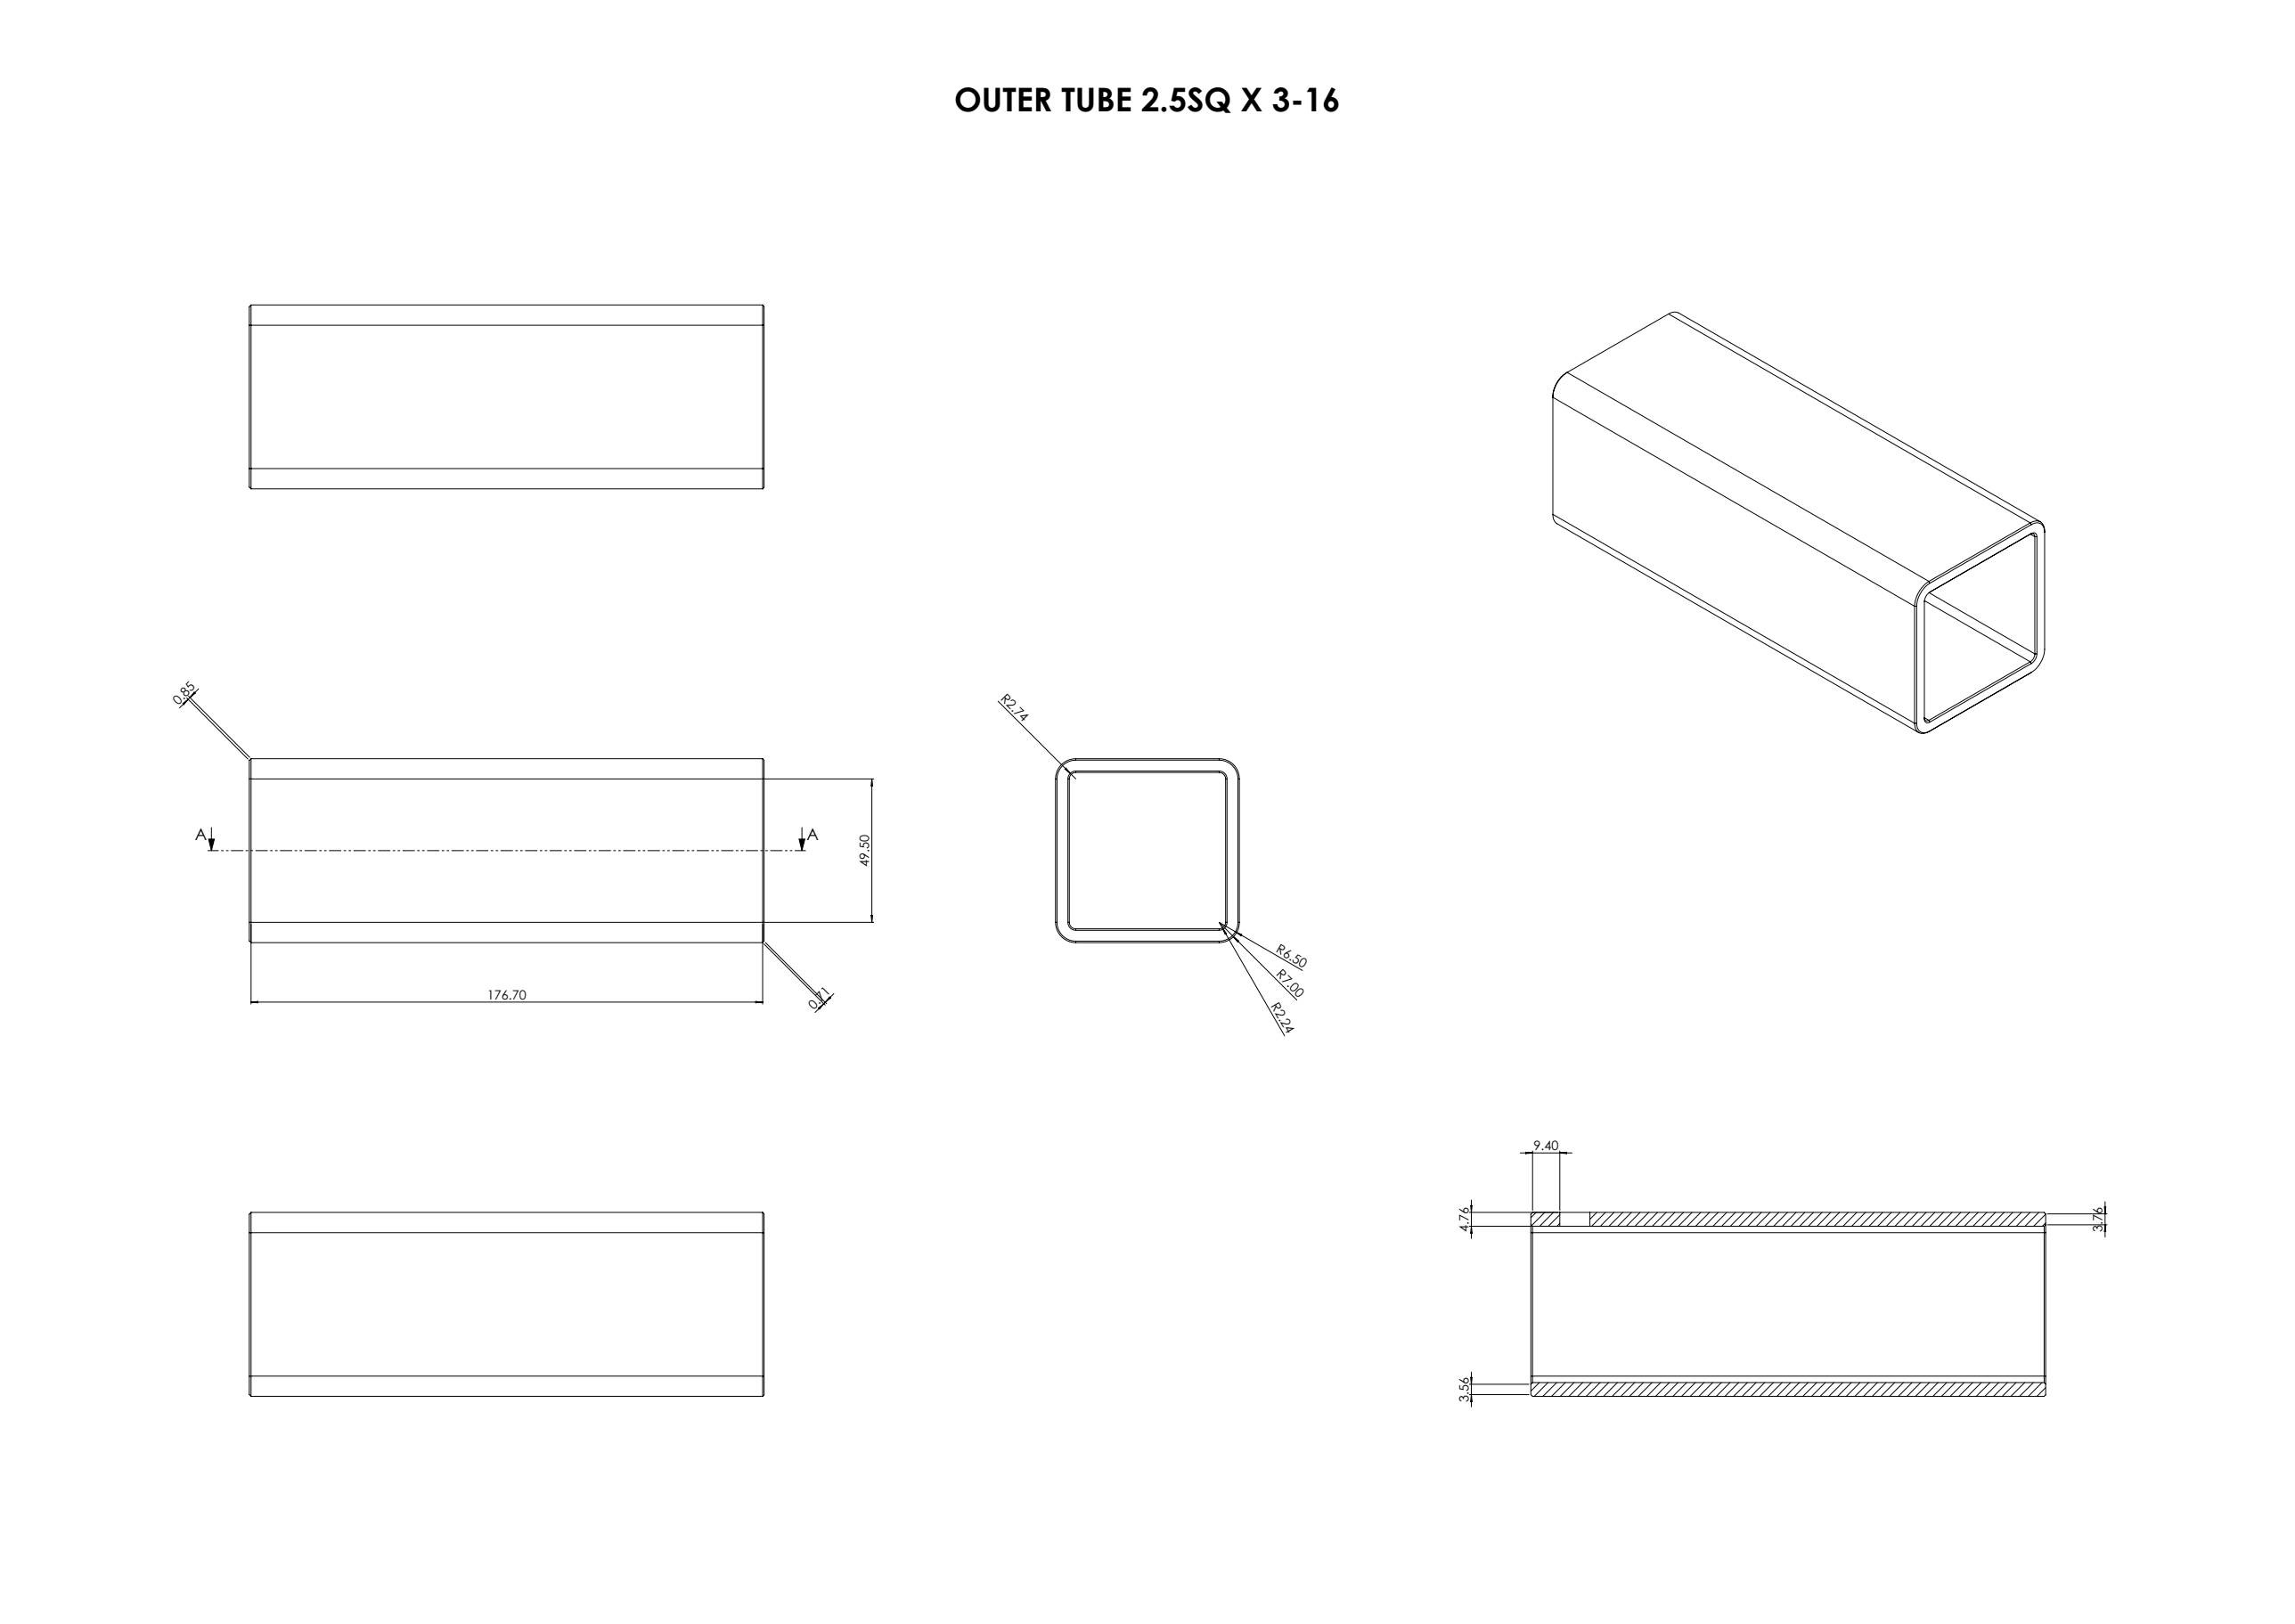
ISO-10303-21;
HEADER;
/* Generated by software containing ST-Developer
 * from STEP Tools, Inc. (www.steptools.com) 
 */

FILE_DESCRIPTION(
/* description */ (''),
/* implementation_level */ '2;1');

FILE_NAME(
/* name */ '01_Outer_Tube_2.5sq_x_3-16.step',
/* time_stamp */ '2026-10-25T01:30:15-07:00',
/* author */ (''),
/* organization */ (''),
/* preprocessor_version */ 'ST-DEVELOPER v20.2',
/* originating_system */ 'Autodesk Translation Framework v15.15.0.0',
/* authorisation */ '');

FILE_SCHEMA (('AUTOMOTIVE_DESIGN { 1 0 10303 214 3 1 1 }'));
ENDSEC;

DATA;
#10=MECHANICAL_DESIGN_GEOMETRIC_PRESENTATION_REPRESENTATION('',(#563),#32309);
#535=SHAPE_REPRESENTATION_RELATIONSHIP('SRR','None',#32362,#549);
#549=ADVANCED_BREP_SHAPE_REPRESENTATION('',(#577),#32295);
#563=STYLED_ITEM('',(#32488),#577);
#577=MANIFOLD_SOLID_BREP('Body1',#13804);
#591=FACE_BOUND('',#2051,.T.);
#592=FACE_BOUND('',#2055,.T.);
#593=FACE_BOUND('',#2078,.T.);
#594=FACE_BOUND('',#2095,.T.);
#647=CYLINDRICAL_SURFACE('',#13991,2.2375);
#648=CYLINDRICAL_SURFACE('',#13995,2.23749999999999);
#649=CYLINDRICAL_SURFACE('',#14015,7.);
#650=CYLINDRICAL_SURFACE('',#14018,7.);
#651=CYLINDRICAL_SURFACE('',#14035,7.);
#652=CYLINDRICAL_SURFACE('',#14051,2.23749999999998);
#653=CYLINDRICAL_SURFACE('',#14052,5.2);
#654=CYLINDRICAL_SURFACE('',#14055,2.2375);
#655=CYLINDRICAL_SURFACE('',#14058,7.);
#773=CIRCLE('',#13977,2.73749999999998);
#774=CIRCLE('',#13978,2.23749999999999);
#775=CIRCLE('',#13981,2.7375);
#776=CIRCLE('',#13982,2.2375);
#777=CIRCLE('',#13985,2.7375);
#778=CIRCLE('',#13986,2.2375);
#779=CIRCLE('',#13989,2.73749999999998);
#780=CIRCLE('',#13990,2.23749999999998);
#781=CIRCLE('',#13992,2.2375);
#782=CIRCLE('',#13994,5.2);
#783=CIRCLE('',#13996,2.23749999999999);
#784=CIRCLE('',#13999,6.5);
#785=CIRCLE('',#14000,6.5);
#786=CIRCLE('',#14001,6.50000000000001);
#787=CIRCLE('',#14002,6.5);
#788=CIRCLE('',#14005,7.);
#789=CIRCLE('',#14008,7.);
#790=CIRCLE('',#14011,7.);
#791=CIRCLE('',#14014,7.);
#792=CIRCLE('',#14016,7.);
#793=CIRCLE('',#14019,7.);
#794=CIRCLE('',#14023,6.4);
#795=CIRCLE('',#14026,7.);
#796=CIRCLE('',#14027,6.40000000000001);
#797=CIRCLE('',#14030,7.);
#798=CIRCLE('',#14031,6.40000000000001);
#799=CIRCLE('',#14034,6.4);
#800=CIRCLE('',#14037,2.83749999999998);
#801=CIRCLE('',#14038,2.83749999999998);
#802=CIRCLE('',#14039,2.83750000000001);
#803=CIRCLE('',#14040,2.8375);
#804=CIRCLE('',#14045,2.2375);
#805=CIRCLE('',#14048,2.23749999999998);
#806=CIRCLE('',#14053,5.2);
#1097=CONICAL_SURFACE('',#13976,2.48749999999999,0.785398163397441);
#1098=CONICAL_SURFACE('',#13980,2.4875,0.785398163397441);
#1099=CONICAL_SURFACE('',#13984,2.4875,0.785398163397441);
#1100=CONICAL_SURFACE('',#13988,2.48749999999998,0.785398163397441);
#1101=CONICAL_SURFACE('',#14004,6.75,0.785398163397441);
#1102=CONICAL_SURFACE('',#14007,6.75,0.785398163397441);
#1103=CONICAL_SURFACE('',#14010,6.75000000000001,0.785398163397431);
#1104=CONICAL_SURFACE('',#14013,6.75,0.785398163397441);
#1105=CONICAL_SURFACE('',#14022,6.7,0.78539816339745);
#1106=CONICAL_SURFACE('',#14025,6.70000000000001,0.785398163397438);
#1107=CONICAL_SURFACE('',#14029,6.7,0.785398163397445);
#1108=CONICAL_SURFACE('',#14033,6.7,0.78539816339745);
#1109=CONICAL_SURFACE('',#14042,2.5375,0.78539816339745);
#1110=CONICAL_SURFACE('',#14044,2.5375,0.78539816339745);
#1111=CONICAL_SURFACE('',#14047,2.53749999999998,0.785398163397445);
#1112=CONICAL_SURFACE('',#14050,2.53749999999998,0.785398163397445);
#1242=FACE_OUTER_BOUND('',#2041,.T.);
#1243=FACE_OUTER_BOUND('',#2042,.T.);
#1244=FACE_OUTER_BOUND('',#2043,.T.);
#1245=FACE_OUTER_BOUND('',#2044,.T.);
#1246=FACE_OUTER_BOUND('',#2045,.T.);
#1247=FACE_OUTER_BOUND('',#2046,.T.);
#1248=FACE_OUTER_BOUND('',#2047,.T.);
#1249=FACE_OUTER_BOUND('',#2048,.T.);
#1250=FACE_OUTER_BOUND('',#2049,.T.);
#1251=FACE_OUTER_BOUND('',#2050,.T.);
#1252=FACE_OUTER_BOUND('',#2052,.T.);
#1253=FACE_OUTER_BOUND('',#2053,.T.);
#1254=FACE_OUTER_BOUND('',#2054,.T.);
#1255=FACE_OUTER_BOUND('',#2056,.T.);
#1256=FACE_OUTER_BOUND('',#2057,.T.);
#1257=FACE_OUTER_BOUND('',#2058,.T.);
#1258=FACE_OUTER_BOUND('',#2059,.T.);
#1259=FACE_OUTER_BOUND('',#2060,.T.);
#1260=FACE_OUTER_BOUND('',#2061,.T.);
#1261=FACE_OUTER_BOUND('',#2062,.T.);
#1262=FACE_OUTER_BOUND('',#2063,.T.);
#1263=FACE_OUTER_BOUND('',#2064,.T.);
#1264=FACE_OUTER_BOUND('',#2065,.T.);
#1265=FACE_OUTER_BOUND('',#2066,.T.);
#1266=FACE_OUTER_BOUND('',#2067,.T.);
#1267=FACE_OUTER_BOUND('',#2068,.T.);
#1268=FACE_OUTER_BOUND('',#2069,.T.);
#1269=FACE_OUTER_BOUND('',#2070,.T.);
#1270=FACE_OUTER_BOUND('',#2071,.T.);
#1271=FACE_OUTER_BOUND('',#2072,.T.);
#1272=FACE_OUTER_BOUND('',#2073,.T.);
#1273=FACE_OUTER_BOUND('',#2074,.T.);
#1274=FACE_OUTER_BOUND('',#2075,.T.);
#1275=FACE_OUTER_BOUND('',#2076,.T.);
#1276=FACE_OUTER_BOUND('',#2077,.T.);
#1277=FACE_OUTER_BOUND('',#2079,.T.);
#1278=FACE_OUTER_BOUND('',#2080,.T.);
#1279=FACE_OUTER_BOUND('',#2081,.T.);
#1280=FACE_OUTER_BOUND('',#2082,.T.);
#1281=FACE_OUTER_BOUND('',#2083,.T.);
#1282=FACE_OUTER_BOUND('',#2084,.T.);
#1283=FACE_OUTER_BOUND('',#2085,.T.);
#1284=FACE_OUTER_BOUND('',#2086,.T.);
#1285=FACE_OUTER_BOUND('',#2087,.T.);
#1286=FACE_OUTER_BOUND('',#2088,.T.);
#1287=FACE_OUTER_BOUND('',#2089,.T.);
#1288=FACE_OUTER_BOUND('',#2090,.T.);
#1289=FACE_OUTER_BOUND('',#2091,.T.);
#1290=FACE_OUTER_BOUND('',#2092,.T.);
#1291=FACE_OUTER_BOUND('',#2093,.T.);
#1292=FACE_OUTER_BOUND('',#2094,.T.);
#2041=EDGE_LOOP('',(#8679,#8680,#8681,#8682));
#2042=EDGE_LOOP('',(#8683,#8684,#8685,#8686));
#2043=EDGE_LOOP('',(#8687,#8688,#8689,#8690));
#2044=EDGE_LOOP('',(#8691,#8692,#8693,#8694));
#2045=EDGE_LOOP('',(#8695,#8696,#8697,#8698));
#2046=EDGE_LOOP('',(#8699,#8700,#8701,#8702));
#2047=EDGE_LOOP('',(#8703,#8704,#8705,#8706));
#2048=EDGE_LOOP('',(#8707,#8708,#8709,#8710));
#2049=EDGE_LOOP('',(#8711,#8712,#8713,#8714));
#2050=EDGE_LOOP('',(#8715,#8716,#8717,#8718));
#2051=EDGE_LOOP('',(#8719));
#2052=EDGE_LOOP('',(#8720,#8721,#8722,#8723));
#2053=EDGE_LOOP('',(#8724,#8725,#8726,#8727));
#2054=EDGE_LOOP('',(#8728,#8729,#8730,#8731,#8732,#8733,#8734,#8735));
#2055=EDGE_LOOP('',(#8736,#8737,#8738,#8739,#8740,#8741,#8742,#8743));
#2056=EDGE_LOOP('',(#8744,#8745,#8746,#8747));
#2057=EDGE_LOOP('',(#8748,#8749,#8750,#8751));
#2058=EDGE_LOOP('',(#8752,#8753,#8754,#8755));
#2059=EDGE_LOOP('',(#8756,#8757,#8758,#8759));
#2060=EDGE_LOOP('',(#8760,#8761,#8762,#8763));
#2061=EDGE_LOOP('',(#8764,#8765,#8766,#8767));
#2062=EDGE_LOOP('',(#8768,#8769,#8770,#8771));
#2063=EDGE_LOOP('',(#8772,#8773,#8774,#8775));
#2064=EDGE_LOOP('',(#8776,#8777,#8778,#8779));
#2065=EDGE_LOOP('',(#8780,#8781,#8782,#8783));
#2066=EDGE_LOOP('',(#8784,#8785,#8786,#8787));
#2067=EDGE_LOOP('',(#8788,#8789,#8790,#8791));
#2068=EDGE_LOOP('',(#8792,#8793,#8794,#8795));
#2069=EDGE_LOOP('',(#8796,#8797,#8798,#8799));
#2070=EDGE_LOOP('',(#8800,#8801,#8802,#8803));
#2071=EDGE_LOOP('',(#8804,#8805,#8806,#8807));
#2072=EDGE_LOOP('',(#8808,#8809,#8810,#8811));
#2073=EDGE_LOOP('',(#8812,#8813,#8814,#8815));
#2074=EDGE_LOOP('',(#8816,#8817,#8818,#8819));
#2075=EDGE_LOOP('',(#8820,#8821,#8822,#8823));
#2076=EDGE_LOOP('',(#8824,#8825,#8826,#8827));
#2077=EDGE_LOOP('',(#8828,#8829,#8830,#8831,#8832,#8833,#8834,#8835));
#2078=EDGE_LOOP('',(#8836,#8837,#8838,#8839,#8840,#8841,#8842,#8843));
#2079=EDGE_LOOP('',(#8844,#8845,#8846,#8847));
#2080=EDGE_LOOP('',(#8848,#8849,#8850,#8851));
#2081=EDGE_LOOP('',(#8852,#8853,#8854,#8855));
#2082=EDGE_LOOP('',(#8856,#8857,#8858,#8859));
#2083=EDGE_LOOP('',(#8860,#8861,#8862,#8863));
#2084=EDGE_LOOP('',(#8864,#8865,#8866,#8867));
#2085=EDGE_LOOP('',(#8868,#8869,#8870,#8871));
#2086=EDGE_LOOP('',(#8872,#8873,#8874,#8875));
#2087=EDGE_LOOP('',(#8876,#8877,#8878,#8879));
#2088=EDGE_LOOP('',(#8880,#8881,#8882,#8883));
#2089=EDGE_LOOP('',(#8884,#8885,#8886,#8887));
#2090=EDGE_LOOP('',(#8888,#8889,#8890,#8891));
#2091=EDGE_LOOP('',(#8892,#8893,#8894,#8895));
#2092=EDGE_LOOP('',(#8896,#8897,#8898,#8899));
#2093=EDGE_LOOP('',(#8900,#8901,#8902,#8903));
#2094=EDGE_LOOP('',(#8904,#8905,#8906,#8907));
#2095=EDGE_LOOP('',(#8908));
#2896=LINE('',#18382,#4207);
#2897=LINE('',#18384,#4208);
#2898=LINE('',#18386,#4209);
#2899=LINE('',#18387,#4210);
#2900=LINE('',#18391,#4211);
#2901=LINE('',#18397,#4212);
#2902=LINE('',#18398,#4213);
#2903=LINE('',#18399,#4214);
#2904=LINE('',#18403,#4215);
#2905=LINE('',#18409,#4216);
#2906=LINE('',#18410,#4217);
#2907=LINE('',#18411,#4218);
#2908=LINE('',#18415,#4219);
#2909=LINE('',#18421,#4220);
#2910=LINE('',#18422,#4221);
#2911=LINE('',#18423,#4222);
#2912=LINE('',#18429,#4223);
#2913=LINE('',#18432,#4224);
#2914=LINE('',#18435,#4225);
#2915=LINE('',#18436,#4226);
#2916=LINE('',#18441,#4227);
#2917=LINE('',#18445,#4228);
#2918=LINE('',#18446,#4229);
#2919=LINE('',#18450,#4230);
#2920=LINE('',#18454,#4231);
#2921=LINE('',#18458,#4232);
#2922=LINE('',#18462,#4233);
#2923=LINE('',#18466,#4234);
#2924=LINE('',#18468,#4235);
#2925=LINE('',#18469,#4236);
#2926=LINE('',#18472,#4237);
#2927=LINE('',#18476,#4238);
#2928=LINE('',#18477,#4239);
#2929=LINE('',#18480,#4240);
#2930=LINE('',#18484,#4241);
#2931=LINE('',#18485,#4242);
#2932=LINE('',#18488,#4243);
#2933=LINE('',#18492,#4244);
#2934=LINE('',#18493,#4245);
#2935=LINE('',#18498,#4246);
#2936=LINE('',#18501,#4247);
#2937=LINE('',#18504,#4248);
#2938=LINE('',#18505,#4249);
#2939=LINE('',#18508,#4250);
#2940=LINE('',#18512,#4251);
#2941=LINE('',#18513,#4252);
#2942=LINE('',#18516,#4253);
#2943=LINE('',#18518,#4254);
#2944=LINE('',#18519,#4255);
#2945=LINE('',#18522,#4256);
#2946=LINE('',#18527,#4257);
#2947=LINE('',#18528,#4258);
#2948=LINE('',#18529,#4259);
#2949=LINE('',#18533,#4260);
#2950=LINE('',#18539,#4261);
#2951=LINE('',#18540,#4262);
#2952=LINE('',#18541,#4263);
#2953=LINE('',#18544,#4264);
#2954=LINE('',#18549,#4265);
#2955=LINE('',#18550,#4266);
#2956=LINE('',#18554,#4267);
#2957=LINE('',#18558,#4268);
#2958=LINE('',#18562,#4269);
#2959=LINE('',#18566,#4270);
#2960=LINE('',#18570,#4271);
#2961=LINE('',#18573,#4272);
#2962=LINE('',#18574,#4273);
#2963=LINE('',#18576,#4274);
#2964=LINE('',#18579,#4275);
#2965=LINE('',#18580,#4276);
#2966=LINE('',#18583,#4277);
#2967=LINE('',#18587,#4278);
#2968=LINE('',#18588,#4279);
#2969=LINE('',#18590,#4280);
#2970=LINE('',#18593,#4281);
#2971=LINE('',#18596,#4282);
#2972=LINE('',#18600,#4283);
#2973=LINE('',#18602,#4284);
#2974=LINE('',#18604,#4285);
#2975=LINE('',#18607,#4286);
#2976=LINE('',#18609,#4287);
#4207=VECTOR('',#15010,10.);
#4208=VECTOR('',#15011,10.);
#4209=VECTOR('',#15012,10.);
#4210=VECTOR('',#15013,10.);
#4211=VECTOR('',#15016,10.);
#4212=VECTOR('',#15023,10.);
#4213=VECTOR('',#15024,10.);
#4214=VECTOR('',#15025,10.);
#4215=VECTOR('',#15028,10.);
#4216=VECTOR('',#15035,10.);
#4217=VECTOR('',#15036,10.);
#4218=VECTOR('',#15037,10.);
#4219=VECTOR('',#15040,10.);
#4220=VECTOR('',#15047,10.);
#4221=VECTOR('',#15048,10.);
#4222=VECTOR('',#15049,10.);
#4223=VECTOR('',#15058,10.);
#4224=VECTOR('',#15061,10.);
#4225=VECTOR('',#15064,10.);
#4226=VECTOR('',#15065,10.);
#4227=VECTOR('',#15070,10.);
#4228=VECTOR('',#15075,10.);
#4229=VECTOR('',#15076,10.);
#4230=VECTOR('',#15079,10.);
#4231=VECTOR('',#15082,10.);
#4232=VECTOR('',#15085,10.);
#4233=VECTOR('',#15088,10.);
#4234=VECTOR('',#15093,10.);
#4235=VECTOR('',#15094,10.);
#4236=VECTOR('',#15095,10.);
#4237=VECTOR('',#15098,10.);
#4238=VECTOR('',#15103,10.);
#4239=VECTOR('',#15104,10.);
#4240=VECTOR('',#15107,10.);
#4241=VECTOR('',#15112,10.);
#4242=VECTOR('',#15113,10.);
#4243=VECTOR('',#15116,10.);
#4244=VECTOR('',#15121,10.);
#4245=VECTOR('',#15122,10.);
#4246=VECTOR('',#15129,10.);
#4247=VECTOR('',#15132,10.);
#4248=VECTOR('',#15135,10.);
#4249=VECTOR('',#15136,10.);
#4250=VECTOR('',#15139,10.);
#4251=VECTOR('',#15144,10.);
#4252=VECTOR('',#15145,10.);
#4253=VECTOR('',#15148,10.);
#4254=VECTOR('',#15149,10.);
#4255=VECTOR('',#15150,10.);
#4256=VECTOR('',#15153,10.);
#4257=VECTOR('',#15158,10.);
#4258=VECTOR('',#15159,10.);
#4259=VECTOR('',#15160,10.);
#4260=VECTOR('',#15163,10.);
#4261=VECTOR('',#15170,10.);
#4262=VECTOR('',#15171,10.);
#4263=VECTOR('',#15172,10.);
#4264=VECTOR('',#15175,10.);
#4265=VECTOR('',#15182,10.);
#4266=VECTOR('',#15183,10.);
#4267=VECTOR('',#15190,10.);
#4268=VECTOR('',#15193,10.);
#4269=VECTOR('',#15196,10.);
#4270=VECTOR('',#15199,10.);
#4271=VECTOR('',#15202,10.);
#4272=VECTOR('',#15207,10.);
#4273=VECTOR('',#15208,10.);
#4274=VECTOR('',#15211,10.);
#4275=VECTOR('',#15214,10.);
#4276=VECTOR('',#15215,10.);
#4277=VECTOR('',#15218,10.);
#4278=VECTOR('',#15223,10.);
#4279=VECTOR('',#15224,10.);
#4280=VECTOR('',#15227,10.);
#4281=VECTOR('',#15232,10.);
#4282=VECTOR('',#15237,10.);
#4283=VECTOR('',#15242,5.2);
#4284=VECTOR('',#15245,10.);
#4285=VECTOR('',#15248,10.);
#4286=VECTOR('',#15253,10.);
#4287=VECTOR('',#15256,10.);
#5518=VERTEX_POINT('',#18380);
#5519=VERTEX_POINT('',#18381);
#5520=VERTEX_POINT('',#18383);
#5521=VERTEX_POINT('',#18385);
#5522=VERTEX_POINT('',#18389);
#5523=VERTEX_POINT('',#18390);
#5524=VERTEX_POINT('',#18395);
#5525=VERTEX_POINT('',#18396);
#5526=VERTEX_POINT('',#18401);
#5527=VERTEX_POINT('',#18402);
#5528=VERTEX_POINT('',#18407);
#5529=VERTEX_POINT('',#18408);
#5530=VERTEX_POINT('',#18413);
#5531=VERTEX_POINT('',#18414);
#5532=VERTEX_POINT('',#18419);
#5533=VERTEX_POINT('',#18420);
#5534=VERTEX_POINT('',#18428);
#5535=VERTEX_POINT('',#18430);
#5536=VERTEX_POINT('',#18434);
#5537=VERTEX_POINT('',#18437);
#5538=VERTEX_POINT('',#18440);
#5539=VERTEX_POINT('',#18444);
#5540=VERTEX_POINT('',#18448);
#5541=VERTEX_POINT('',#18449);
#5542=VERTEX_POINT('',#18451);
#5543=VERTEX_POINT('',#18453);
#5544=VERTEX_POINT('',#18455);
#5545=VERTEX_POINT('',#18457);
#5546=VERTEX_POINT('',#18459);
#5547=VERTEX_POINT('',#18461);
#5548=VERTEX_POINT('',#18465);
#5549=VERTEX_POINT('',#18467);
#5550=VERTEX_POINT('',#18471);
#5551=VERTEX_POINT('',#18475);
#5552=VERTEX_POINT('',#18479);
#5553=VERTEX_POINT('',#18483);
#5554=VERTEX_POINT('',#18487);
#5555=VERTEX_POINT('',#18491);
#5556=VERTEX_POINT('',#18497);
#5557=VERTEX_POINT('',#18499);
#5558=VERTEX_POINT('',#18503);
#5559=VERTEX_POINT('',#18507);
#5560=VERTEX_POINT('',#18511);
#5561=VERTEX_POINT('',#18515);
#5562=VERTEX_POINT('',#18517);
#5563=VERTEX_POINT('',#18521);
#5564=VERTEX_POINT('',#18525);
#5565=VERTEX_POINT('',#18526);
#5566=VERTEX_POINT('',#18531);
#5567=VERTEX_POINT('',#18532);
#5568=VERTEX_POINT('',#18537);
#5569=VERTEX_POINT('',#18538);
#5570=VERTEX_POINT('',#18543);
#5571=VERTEX_POINT('',#18548);
#5572=VERTEX_POINT('',#18556);
#5573=VERTEX_POINT('',#18557);
#5574=VERTEX_POINT('',#18559);
#5575=VERTEX_POINT('',#18561);
#5576=VERTEX_POINT('',#18563);
#5577=VERTEX_POINT('',#18565);
#5578=VERTEX_POINT('',#18567);
#5579=VERTEX_POINT('',#18569);
#5580=VERTEX_POINT('',#18578);
#5581=VERTEX_POINT('',#18582);
#5582=VERTEX_POINT('',#18586);
#5583=VERTEX_POINT('',#18598);
#6716=EDGE_CURVE('',#5518,#5519,#2896,.T.);
#6717=EDGE_CURVE('',#5519,#5520,#2897,.T.);
#6718=EDGE_CURVE('',#5520,#5521,#2898,.T.);
#6719=EDGE_CURVE('',#5521,#5518,#2899,.T.);
#6720=EDGE_CURVE('',#5522,#5523,#2900,.T.);
#6721=EDGE_CURVE('',#5523,#5519,#773,.T.);
#6722=EDGE_CURVE('',#5518,#5522,#774,.T.);
#6723=EDGE_CURVE('',#5524,#5525,#2901,.T.);
#6724=EDGE_CURVE('',#5525,#5523,#2902,.T.);
#6725=EDGE_CURVE('',#5522,#5524,#2903,.T.);
#6726=EDGE_CURVE('',#5526,#5527,#2904,.T.);
#6727=EDGE_CURVE('',#5527,#5525,#775,.T.);
#6728=EDGE_CURVE('',#5524,#5526,#776,.T.);
#6729=EDGE_CURVE('',#5528,#5529,#2905,.T.);
#6730=EDGE_CURVE('',#5529,#5527,#2906,.T.);
#6731=EDGE_CURVE('',#5526,#5528,#2907,.T.);
#6732=EDGE_CURVE('',#5530,#5531,#2908,.T.);
#6733=EDGE_CURVE('',#5531,#5529,#777,.T.);
#6734=EDGE_CURVE('',#5528,#5530,#778,.T.);
#6735=EDGE_CURVE('',#5532,#5533,#2909,.T.);
#6736=EDGE_CURVE('',#5533,#5531,#2910,.T.);
#6737=EDGE_CURVE('',#5530,#5532,#2911,.T.);
#6738=EDGE_CURVE('',#5520,#5533,#779,.T.);
#6739=EDGE_CURVE('',#5532,#5521,#780,.T.);
#6740=EDGE_CURVE('',#5534,#5524,#2912,.T.);
#6741=EDGE_CURVE('',#5535,#5534,#781,.T.);
#6742=EDGE_CURVE('',#5535,#5526,#2913,.T.);
#6743=EDGE_CURVE('',#5536,#5522,#2914,.T.);
#6744=EDGE_CURVE('',#5534,#5536,#2915,.T.);
#6745=EDGE_CURVE('',#5537,#5537,#782,.T.);
#6746=EDGE_CURVE('',#5538,#5518,#2916,.T.);
#6747=EDGE_CURVE('',#5536,#5538,#783,.T.);
#6748=EDGE_CURVE('',#5539,#5521,#2917,.T.);
#6749=EDGE_CURVE('',#5538,#5539,#2918,.T.);
#6750=EDGE_CURVE('',#5540,#5541,#2919,.T.);
#6751=EDGE_CURVE('',#5542,#5540,#784,.T.);
#6752=EDGE_CURVE('',#5543,#5542,#2920,.T.);
#6753=EDGE_CURVE('',#5544,#5543,#785,.T.);
#6754=EDGE_CURVE('',#5545,#5544,#2921,.T.);
#6755=EDGE_CURVE('',#5546,#5545,#786,.T.);
#6756=EDGE_CURVE('',#5547,#5546,#2922,.T.);
#6757=EDGE_CURVE('',#5541,#5547,#787,.T.);
#6758=EDGE_CURVE('',#5548,#5540,#2923,.T.);
#6759=EDGE_CURVE('',#5541,#5549,#2924,.T.);
#6760=EDGE_CURVE('',#5549,#5548,#2925,.T.);
#6761=EDGE_CURVE('',#5550,#5542,#2926,.T.);
#6762=EDGE_CURVE('',#5548,#5550,#788,.T.);
#6763=EDGE_CURVE('',#5551,#5543,#2927,.T.);
#6764=EDGE_CURVE('',#5550,#5551,#2928,.T.);
#6765=EDGE_CURVE('',#5552,#5544,#2929,.T.);
#6766=EDGE_CURVE('',#5551,#5552,#789,.T.);
#6767=EDGE_CURVE('',#5553,#5545,#2930,.T.);
#6768=EDGE_CURVE('',#5552,#5553,#2931,.T.);
#6769=EDGE_CURVE('',#5554,#5546,#2932,.T.);
#6770=EDGE_CURVE('',#5553,#5554,#790,.T.);
#6771=EDGE_CURVE('',#5555,#5547,#2933,.T.);
#6772=EDGE_CURVE('',#5554,#5555,#2934,.T.);
#6773=EDGE_CURVE('',#5555,#5549,#791,.T.);
#6774=EDGE_CURVE('',#5556,#5551,#2935,.T.);
#6775=EDGE_CURVE('',#5557,#5556,#792,.T.);
#6776=EDGE_CURVE('',#5557,#5552,#2936,.T.);
#6777=EDGE_CURVE('',#5558,#5550,#2937,.T.);
#6778=EDGE_CURVE('',#5556,#5558,#2938,.T.);
#6779=EDGE_CURVE('',#5559,#5548,#2939,.T.);
#6780=EDGE_CURVE('',#5558,#5559,#793,.T.);
#6781=EDGE_CURVE('',#5560,#5549,#2940,.T.);
#6782=EDGE_CURVE('',#5559,#5560,#2941,.T.);
#6783=EDGE_CURVE('',#5561,#5556,#2942,.T.);
#6784=EDGE_CURVE('',#5558,#5562,#2943,.T.);
#6785=EDGE_CURVE('',#5562,#5561,#2944,.T.);
#6786=EDGE_CURVE('',#5563,#5557,#2945,.T.);
#6787=EDGE_CURVE('',#5561,#5563,#794,.T.);
#6788=EDGE_CURVE('',#5564,#5565,#2946,.T.);
#6789=EDGE_CURVE('',#5565,#5557,#2947,.T.);
#6790=EDGE_CURVE('',#5563,#5564,#2948,.T.);
#6791=EDGE_CURVE('',#5566,#5567,#2949,.T.);
#6792=EDGE_CURVE('',#5567,#5565,#795,.T.);
#6793=EDGE_CURVE('',#5564,#5566,#796,.T.);
#6794=EDGE_CURVE('',#5568,#5569,#2950,.T.);
#6795=EDGE_CURVE('',#5569,#5567,#2951,.T.);
#6796=EDGE_CURVE('',#5566,#5568,#2952,.T.);
#6797=EDGE_CURVE('',#5570,#5560,#2953,.T.);
#6798=EDGE_CURVE('',#5560,#5569,#797,.T.);
#6799=EDGE_CURVE('',#5568,#5570,#798,.T.);
#6800=EDGE_CURVE('',#5571,#5559,#2954,.T.);
#6801=EDGE_CURVE('',#5570,#5571,#2955,.T.);
#6802=EDGE_CURVE('',#5571,#5562,#799,.T.);
#6803=EDGE_CURVE('',#5569,#5555,#2956,.T.);
#6804=EDGE_CURVE('',#5572,#5573,#2957,.T.);
#6805=EDGE_CURVE('',#5574,#5572,#800,.T.);
#6806=EDGE_CURVE('',#5575,#5574,#2958,.T.);
#6807=EDGE_CURVE('',#5576,#5575,#801,.T.);
#6808=EDGE_CURVE('',#5577,#5576,#2959,.T.);
#6809=EDGE_CURVE('',#5578,#5577,#802,.T.);
#6810=EDGE_CURVE('',#5579,#5578,#2960,.T.);
#6811=EDGE_CURVE('',#5573,#5579,#803,.T.);
#6812=EDGE_CURVE('',#5573,#5534,#2961,.T.);
#6813=EDGE_CURVE('',#5536,#5572,#2962,.T.);
#6814=EDGE_CURVE('',#5579,#5535,#2963,.T.);
#6815=EDGE_CURVE('',#5578,#5580,#2964,.T.);
#6816=EDGE_CURVE('',#5580,#5535,#2965,.T.);
#6817=EDGE_CURVE('',#5577,#5581,#2966,.T.);
#6818=EDGE_CURVE('',#5581,#5580,#804,.T.);
#6819=EDGE_CURVE('',#5576,#5582,#2967,.T.);
#6820=EDGE_CURVE('',#5582,#5581,#2968,.T.);
#6821=EDGE_CURVE('',#5575,#5539,#2969,.T.);
#6822=EDGE_CURVE('',#5539,#5582,#805,.T.);
#6823=EDGE_CURVE('',#5574,#5538,#2970,.T.);
#6824=EDGE_CURVE('',#5582,#5532,#2971,.T.);
#6825=EDGE_CURVE('',#5583,#5583,#806,.T.);
#6826=EDGE_CURVE('',#5583,#5537,#2972,.T.);
#6827=EDGE_CURVE('',#5581,#5530,#2973,.T.);
#6828=EDGE_CURVE('',#5580,#5528,#2974,.T.);
#6829=EDGE_CURVE('',#5567,#5554,#2975,.T.);
#6830=EDGE_CURVE('',#5565,#5553,#2976,.T.);
#8679=ORIENTED_EDGE('',*,*,#6716,.T.);
#8680=ORIENTED_EDGE('',*,*,#6717,.T.);
#8681=ORIENTED_EDGE('',*,*,#6718,.T.);
#8682=ORIENTED_EDGE('',*,*,#6719,.T.);
#8683=ORIENTED_EDGE('',*,*,#6720,.T.);
#8684=ORIENTED_EDGE('',*,*,#6721,.T.);
#8685=ORIENTED_EDGE('',*,*,#6716,.F.);
#8686=ORIENTED_EDGE('',*,*,#6722,.T.);
#8687=ORIENTED_EDGE('',*,*,#6723,.T.);
#8688=ORIENTED_EDGE('',*,*,#6724,.T.);
#8689=ORIENTED_EDGE('',*,*,#6720,.F.);
#8690=ORIENTED_EDGE('',*,*,#6725,.T.);
#8691=ORIENTED_EDGE('',*,*,#6726,.T.);
#8692=ORIENTED_EDGE('',*,*,#6727,.T.);
#8693=ORIENTED_EDGE('',*,*,#6723,.F.);
#8694=ORIENTED_EDGE('',*,*,#6728,.T.);
#8695=ORIENTED_EDGE('',*,*,#6729,.T.);
#8696=ORIENTED_EDGE('',*,*,#6730,.T.);
#8697=ORIENTED_EDGE('',*,*,#6726,.F.);
#8698=ORIENTED_EDGE('',*,*,#6731,.T.);
#8699=ORIENTED_EDGE('',*,*,#6732,.T.);
#8700=ORIENTED_EDGE('',*,*,#6733,.T.);
#8701=ORIENTED_EDGE('',*,*,#6729,.F.);
#8702=ORIENTED_EDGE('',*,*,#6734,.T.);
#8703=ORIENTED_EDGE('',*,*,#6735,.T.);
#8704=ORIENTED_EDGE('',*,*,#6736,.T.);
#8705=ORIENTED_EDGE('',*,*,#6732,.F.);
#8706=ORIENTED_EDGE('',*,*,#6737,.T.);
#8707=ORIENTED_EDGE('',*,*,#6718,.F.);
#8708=ORIENTED_EDGE('',*,*,#6738,.T.);
#8709=ORIENTED_EDGE('',*,*,#6735,.F.);
#8710=ORIENTED_EDGE('',*,*,#6739,.T.);
#8711=ORIENTED_EDGE('',*,*,#6728,.F.);
#8712=ORIENTED_EDGE('',*,*,#6740,.F.);
#8713=ORIENTED_EDGE('',*,*,#6741,.F.);
#8714=ORIENTED_EDGE('',*,*,#6742,.T.);
#8715=ORIENTED_EDGE('',*,*,#6725,.F.);
#8716=ORIENTED_EDGE('',*,*,#6743,.F.);
#8717=ORIENTED_EDGE('',*,*,#6744,.F.);
#8718=ORIENTED_EDGE('',*,*,#6740,.T.);
#8719=ORIENTED_EDGE('',*,*,#6745,.T.);
#8720=ORIENTED_EDGE('',*,*,#6722,.F.);
#8721=ORIENTED_EDGE('',*,*,#6746,.F.);
#8722=ORIENTED_EDGE('',*,*,#6747,.F.);
#8723=ORIENTED_EDGE('',*,*,#6743,.T.);
#8724=ORIENTED_EDGE('',*,*,#6719,.F.);
#8725=ORIENTED_EDGE('',*,*,#6748,.F.);
#8726=ORIENTED_EDGE('',*,*,#6749,.F.);
#8727=ORIENTED_EDGE('',*,*,#6746,.T.);
#8728=ORIENTED_EDGE('',*,*,#6750,.F.);
#8729=ORIENTED_EDGE('',*,*,#6751,.F.);
#8730=ORIENTED_EDGE('',*,*,#6752,.F.);
#8731=ORIENTED_EDGE('',*,*,#6753,.F.);
#8732=ORIENTED_EDGE('',*,*,#6754,.F.);
#8733=ORIENTED_EDGE('',*,*,#6755,.F.);
#8734=ORIENTED_EDGE('',*,*,#6756,.F.);
#8735=ORIENTED_EDGE('',*,*,#6757,.F.);
#8736=ORIENTED_EDGE('',*,*,#6717,.F.);
#8737=ORIENTED_EDGE('',*,*,#6721,.F.);
#8738=ORIENTED_EDGE('',*,*,#6724,.F.);
#8739=ORIENTED_EDGE('',*,*,#6727,.F.);
#8740=ORIENTED_EDGE('',*,*,#6730,.F.);
#8741=ORIENTED_EDGE('',*,*,#6733,.F.);
#8742=ORIENTED_EDGE('',*,*,#6736,.F.);
#8743=ORIENTED_EDGE('',*,*,#6738,.F.);
#8744=ORIENTED_EDGE('',*,*,#6758,.T.);
#8745=ORIENTED_EDGE('',*,*,#6750,.T.);
#8746=ORIENTED_EDGE('',*,*,#6759,.T.);
#8747=ORIENTED_EDGE('',*,*,#6760,.T.);
#8748=ORIENTED_EDGE('',*,*,#6761,.T.);
#8749=ORIENTED_EDGE('',*,*,#6751,.T.);
#8750=ORIENTED_EDGE('',*,*,#6758,.F.);
#8751=ORIENTED_EDGE('',*,*,#6762,.T.);
#8752=ORIENTED_EDGE('',*,*,#6763,.T.);
#8753=ORIENTED_EDGE('',*,*,#6752,.T.);
#8754=ORIENTED_EDGE('',*,*,#6761,.F.);
#8755=ORIENTED_EDGE('',*,*,#6764,.T.);
#8756=ORIENTED_EDGE('',*,*,#6765,.T.);
#8757=ORIENTED_EDGE('',*,*,#6753,.T.);
#8758=ORIENTED_EDGE('',*,*,#6763,.F.);
#8759=ORIENTED_EDGE('',*,*,#6766,.T.);
#8760=ORIENTED_EDGE('',*,*,#6767,.T.);
#8761=ORIENTED_EDGE('',*,*,#6754,.T.);
#8762=ORIENTED_EDGE('',*,*,#6765,.F.);
#8763=ORIENTED_EDGE('',*,*,#6768,.T.);
#8764=ORIENTED_EDGE('',*,*,#6769,.T.);
#8765=ORIENTED_EDGE('',*,*,#6755,.T.);
#8766=ORIENTED_EDGE('',*,*,#6767,.F.);
#8767=ORIENTED_EDGE('',*,*,#6770,.T.);
#8768=ORIENTED_EDGE('',*,*,#6771,.T.);
#8769=ORIENTED_EDGE('',*,*,#6756,.T.);
#8770=ORIENTED_EDGE('',*,*,#6769,.F.);
#8771=ORIENTED_EDGE('',*,*,#6772,.T.);
#8772=ORIENTED_EDGE('',*,*,#6759,.F.);
#8773=ORIENTED_EDGE('',*,*,#6757,.T.);
#8774=ORIENTED_EDGE('',*,*,#6771,.F.);
#8775=ORIENTED_EDGE('',*,*,#6773,.T.);
#8776=ORIENTED_EDGE('',*,*,#6766,.F.);
#8777=ORIENTED_EDGE('',*,*,#6774,.F.);
#8778=ORIENTED_EDGE('',*,*,#6775,.F.);
#8779=ORIENTED_EDGE('',*,*,#6776,.T.);
#8780=ORIENTED_EDGE('',*,*,#6764,.F.);
#8781=ORIENTED_EDGE('',*,*,#6777,.F.);
#8782=ORIENTED_EDGE('',*,*,#6778,.F.);
#8783=ORIENTED_EDGE('',*,*,#6774,.T.);
#8784=ORIENTED_EDGE('',*,*,#6762,.F.);
#8785=ORIENTED_EDGE('',*,*,#6779,.F.);
#8786=ORIENTED_EDGE('',*,*,#6780,.F.);
#8787=ORIENTED_EDGE('',*,*,#6777,.T.);
#8788=ORIENTED_EDGE('',*,*,#6760,.F.);
#8789=ORIENTED_EDGE('',*,*,#6781,.F.);
#8790=ORIENTED_EDGE('',*,*,#6782,.F.);
#8791=ORIENTED_EDGE('',*,*,#6779,.T.);
#8792=ORIENTED_EDGE('',*,*,#6783,.T.);
#8793=ORIENTED_EDGE('',*,*,#6778,.T.);
#8794=ORIENTED_EDGE('',*,*,#6784,.T.);
#8795=ORIENTED_EDGE('',*,*,#6785,.T.);
#8796=ORIENTED_EDGE('',*,*,#6786,.T.);
#8797=ORIENTED_EDGE('',*,*,#6775,.T.);
#8798=ORIENTED_EDGE('',*,*,#6783,.F.);
#8799=ORIENTED_EDGE('',*,*,#6787,.T.);
#8800=ORIENTED_EDGE('',*,*,#6788,.T.);
#8801=ORIENTED_EDGE('',*,*,#6789,.T.);
#8802=ORIENTED_EDGE('',*,*,#6786,.F.);
#8803=ORIENTED_EDGE('',*,*,#6790,.T.);
#8804=ORIENTED_EDGE('',*,*,#6791,.T.);
#8805=ORIENTED_EDGE('',*,*,#6792,.T.);
#8806=ORIENTED_EDGE('',*,*,#6788,.F.);
#8807=ORIENTED_EDGE('',*,*,#6793,.T.);
#8808=ORIENTED_EDGE('',*,*,#6794,.T.);
#8809=ORIENTED_EDGE('',*,*,#6795,.T.);
#8810=ORIENTED_EDGE('',*,*,#6791,.F.);
#8811=ORIENTED_EDGE('',*,*,#6796,.T.);
#8812=ORIENTED_EDGE('',*,*,#6797,.T.);
#8813=ORIENTED_EDGE('',*,*,#6798,.T.);
#8814=ORIENTED_EDGE('',*,*,#6794,.F.);
#8815=ORIENTED_EDGE('',*,*,#6799,.T.);
#8816=ORIENTED_EDGE('',*,*,#6800,.T.);
#8817=ORIENTED_EDGE('',*,*,#6782,.T.);
#8818=ORIENTED_EDGE('',*,*,#6797,.F.);
#8819=ORIENTED_EDGE('',*,*,#6801,.T.);
#8820=ORIENTED_EDGE('',*,*,#6784,.F.);
#8821=ORIENTED_EDGE('',*,*,#6780,.T.);
#8822=ORIENTED_EDGE('',*,*,#6800,.F.);
#8823=ORIENTED_EDGE('',*,*,#6802,.T.);
#8824=ORIENTED_EDGE('',*,*,#6773,.F.);
#8825=ORIENTED_EDGE('',*,*,#6803,.F.);
#8826=ORIENTED_EDGE('',*,*,#6798,.F.);
#8827=ORIENTED_EDGE('',*,*,#6781,.T.);
#8828=ORIENTED_EDGE('',*,*,#6785,.F.);
#8829=ORIENTED_EDGE('',*,*,#6802,.F.);
#8830=ORIENTED_EDGE('',*,*,#6801,.F.);
#8831=ORIENTED_EDGE('',*,*,#6799,.F.);
#8832=ORIENTED_EDGE('',*,*,#6796,.F.);
#8833=ORIENTED_EDGE('',*,*,#6793,.F.);
#8834=ORIENTED_EDGE('',*,*,#6790,.F.);
#8835=ORIENTED_EDGE('',*,*,#6787,.F.);
#8836=ORIENTED_EDGE('',*,*,#6804,.F.);
#8837=ORIENTED_EDGE('',*,*,#6805,.F.);
#8838=ORIENTED_EDGE('',*,*,#6806,.F.);
#8839=ORIENTED_EDGE('',*,*,#6807,.F.);
#8840=ORIENTED_EDGE('',*,*,#6808,.F.);
#8841=ORIENTED_EDGE('',*,*,#6809,.F.);
#8842=ORIENTED_EDGE('',*,*,#6810,.F.);
#8843=ORIENTED_EDGE('',*,*,#6811,.F.);
#8844=ORIENTED_EDGE('',*,*,#6812,.T.);
#8845=ORIENTED_EDGE('',*,*,#6744,.T.);
#8846=ORIENTED_EDGE('',*,*,#6813,.T.);
#8847=ORIENTED_EDGE('',*,*,#6804,.T.);
#8848=ORIENTED_EDGE('',*,*,#6814,.T.);
#8849=ORIENTED_EDGE('',*,*,#6741,.T.);
#8850=ORIENTED_EDGE('',*,*,#6812,.F.);
#8851=ORIENTED_EDGE('',*,*,#6811,.T.);
#8852=ORIENTED_EDGE('',*,*,#6815,.T.);
#8853=ORIENTED_EDGE('',*,*,#6816,.T.);
#8854=ORIENTED_EDGE('',*,*,#6814,.F.);
#8855=ORIENTED_EDGE('',*,*,#6810,.T.);
#8856=ORIENTED_EDGE('',*,*,#6817,.T.);
#8857=ORIENTED_EDGE('',*,*,#6818,.T.);
#8858=ORIENTED_EDGE('',*,*,#6815,.F.);
#8859=ORIENTED_EDGE('',*,*,#6809,.T.);
#8860=ORIENTED_EDGE('',*,*,#6819,.T.);
#8861=ORIENTED_EDGE('',*,*,#6820,.T.);
#8862=ORIENTED_EDGE('',*,*,#6817,.F.);
#8863=ORIENTED_EDGE('',*,*,#6808,.T.);
#8864=ORIENTED_EDGE('',*,*,#6821,.T.);
#8865=ORIENTED_EDGE('',*,*,#6822,.T.);
#8866=ORIENTED_EDGE('',*,*,#6819,.F.);
#8867=ORIENTED_EDGE('',*,*,#6807,.T.);
#8868=ORIENTED_EDGE('',*,*,#6823,.T.);
#8869=ORIENTED_EDGE('',*,*,#6749,.T.);
#8870=ORIENTED_EDGE('',*,*,#6821,.F.);
#8871=ORIENTED_EDGE('',*,*,#6806,.T.);
#8872=ORIENTED_EDGE('',*,*,#6813,.F.);
#8873=ORIENTED_EDGE('',*,*,#6747,.T.);
#8874=ORIENTED_EDGE('',*,*,#6823,.F.);
#8875=ORIENTED_EDGE('',*,*,#6805,.T.);
#8876=ORIENTED_EDGE('',*,*,#6739,.F.);
#8877=ORIENTED_EDGE('',*,*,#6824,.F.);
#8878=ORIENTED_EDGE('',*,*,#6822,.F.);
#8879=ORIENTED_EDGE('',*,*,#6748,.T.);
#8880=ORIENTED_EDGE('',*,*,#6825,.F.);
#8881=ORIENTED_EDGE('',*,*,#6826,.T.);
#8882=ORIENTED_EDGE('',*,*,#6745,.F.);
#8883=ORIENTED_EDGE('',*,*,#6826,.F.);
#8884=ORIENTED_EDGE('',*,*,#6737,.F.);
#8885=ORIENTED_EDGE('',*,*,#6827,.F.);
#8886=ORIENTED_EDGE('',*,*,#6820,.F.);
#8887=ORIENTED_EDGE('',*,*,#6824,.T.);
#8888=ORIENTED_EDGE('',*,*,#6734,.F.);
#8889=ORIENTED_EDGE('',*,*,#6828,.F.);
#8890=ORIENTED_EDGE('',*,*,#6818,.F.);
#8891=ORIENTED_EDGE('',*,*,#6827,.T.);
#8892=ORIENTED_EDGE('',*,*,#6731,.F.);
#8893=ORIENTED_EDGE('',*,*,#6742,.F.);
#8894=ORIENTED_EDGE('',*,*,#6816,.F.);
#8895=ORIENTED_EDGE('',*,*,#6828,.T.);
#8896=ORIENTED_EDGE('',*,*,#6772,.F.);
#8897=ORIENTED_EDGE('',*,*,#6829,.F.);
#8898=ORIENTED_EDGE('',*,*,#6795,.F.);
#8899=ORIENTED_EDGE('',*,*,#6803,.T.);
#8900=ORIENTED_EDGE('',*,*,#6770,.F.);
#8901=ORIENTED_EDGE('',*,*,#6830,.F.);
#8902=ORIENTED_EDGE('',*,*,#6792,.F.);
#8903=ORIENTED_EDGE('',*,*,#6829,.T.);
#8904=ORIENTED_EDGE('',*,*,#6768,.F.);
#8905=ORIENTED_EDGE('',*,*,#6776,.F.);
#8906=ORIENTED_EDGE('',*,*,#6789,.F.);
#8907=ORIENTED_EDGE('',*,*,#6830,.T.);
#8908=ORIENTED_EDGE('',*,*,#6825,.T.);
#12605=PLANE('',#13975);
#12606=PLANE('',#13979);
#12607=PLANE('',#13983);
#12608=PLANE('',#13987);
#12609=PLANE('',#13993);
#12610=PLANE('',#13997);
#12611=PLANE('',#13998);
#12612=PLANE('',#14003);
#12613=PLANE('',#14006);
#12614=PLANE('',#14009);
#12615=PLANE('',#14012);
#12616=PLANE('',#14017);
#12617=PLANE('',#14020);
#12618=PLANE('',#14021);
#12619=PLANE('',#14024);
#12620=PLANE('',#14028);
#12621=PLANE('',#14032);
#12622=PLANE('',#14036);
#12623=PLANE('',#14041);
#12624=PLANE('',#14043);
#12625=PLANE('',#14046);
#12626=PLANE('',#14049);
#12627=PLANE('',#14054);
#12628=PLANE('',#14056);
#12629=PLANE('',#14057);
#12630=PLANE('',#14059);
#13005=ADVANCED_FACE('',(#1242),#12605,.T.);
#13006=ADVANCED_FACE('',(#1243),#1097,.F.);
#13007=ADVANCED_FACE('',(#1244),#12606,.T.);
#13008=ADVANCED_FACE('',(#1245),#1098,.F.);
#13009=ADVANCED_FACE('',(#1246),#12607,.T.);
#13010=ADVANCED_FACE('',(#1247),#1099,.F.);
#13011=ADVANCED_FACE('',(#1248),#12608,.T.);
#13012=ADVANCED_FACE('',(#1249),#1100,.F.);
#13013=ADVANCED_FACE('',(#1250),#647,.F.);
#13014=ADVANCED_FACE('',(#1251,#591),#12609,.T.);
#13015=ADVANCED_FACE('',(#1252),#648,.F.);
#13016=ADVANCED_FACE('',(#1253),#12610,.T.);
#13017=ADVANCED_FACE('',(#1254,#592),#12611,.T.);
#13018=ADVANCED_FACE('',(#1255),#12612,.T.);
#13019=ADVANCED_FACE('',(#1256),#1101,.T.);
#13020=ADVANCED_FACE('',(#1257),#12613,.T.);
#13021=ADVANCED_FACE('',(#1258),#1102,.T.);
#13022=ADVANCED_FACE('',(#1259),#12614,.T.);
#13023=ADVANCED_FACE('',(#1260),#1103,.T.);
#13024=ADVANCED_FACE('',(#1261),#12615,.T.);
#13025=ADVANCED_FACE('',(#1262),#1104,.T.);
#13026=ADVANCED_FACE('',(#1263),#649,.T.);
#13027=ADVANCED_FACE('',(#1264),#12616,.T.);
#13028=ADVANCED_FACE('',(#1265),#650,.T.);
#13029=ADVANCED_FACE('',(#1266),#12617,.T.);
#13030=ADVANCED_FACE('',(#1267),#12618,.T.);
#13031=ADVANCED_FACE('',(#1268),#1105,.T.);
#13032=ADVANCED_FACE('',(#1269),#12619,.T.);
#13033=ADVANCED_FACE('',(#1270),#1106,.T.);
#13034=ADVANCED_FACE('',(#1271),#12620,.T.);
#13035=ADVANCED_FACE('',(#1272),#1107,.T.);
#13036=ADVANCED_FACE('',(#1273),#12621,.T.);
#13037=ADVANCED_FACE('',(#1274),#1108,.T.);
#13038=ADVANCED_FACE('',(#1275),#651,.T.);
#13039=ADVANCED_FACE('',(#1276,#593),#12622,.F.);
#13040=ADVANCED_FACE('',(#1277),#12623,.T.);
#13041=ADVANCED_FACE('',(#1278),#1109,.F.);
#13042=ADVANCED_FACE('',(#1279),#12624,.T.);
#13043=ADVANCED_FACE('',(#1280),#1110,.F.);
#13044=ADVANCED_FACE('',(#1281),#12625,.T.);
#13045=ADVANCED_FACE('',(#1282),#1111,.F.);
#13046=ADVANCED_FACE('',(#1283),#12626,.T.);
#13047=ADVANCED_FACE('',(#1284),#1112,.F.);
#13048=ADVANCED_FACE('',(#1285),#652,.F.);
#13049=ADVANCED_FACE('',(#1286),#653,.F.);
#13050=ADVANCED_FACE('',(#1287),#12627,.T.);
#13051=ADVANCED_FACE('',(#1288),#654,.F.);
#13052=ADVANCED_FACE('',(#1289),#12628,.T.);
#13053=ADVANCED_FACE('',(#1290),#12629,.T.);
#13054=ADVANCED_FACE('',(#1291),#655,.T.);
#13055=ADVANCED_FACE('',(#1292,#594),#12630,.T.);
#13804=CLOSED_SHELL('',(#13005,#13006,#13007,#13008,#13009,#13010,#13011,
#13012,#13013,#13014,#13015,#13016,#13017,#13018,#13019,#13020,#13021,#13022,
#13023,#13024,#13025,#13026,#13027,#13028,#13029,#13030,#13031,#13032,#13033,
#13034,#13035,#13036,#13037,#13038,#13039,#13040,#13041,#13042,#13043,#13044,
#13045,#13046,#13047,#13048,#13049,#13050,#13051,#13052,#13053,#13054,#13055));
#13974=AXIS2_PLACEMENT_3D('',#18378,#15006,#15007);
#13975=AXIS2_PLACEMENT_3D('',#18379,#15008,#15009);
#13976=AXIS2_PLACEMENT_3D('',#18388,#15014,#15015);
#13977=AXIS2_PLACEMENT_3D('',#18392,#15017,#15018);
#13978=AXIS2_PLACEMENT_3D('',#18393,#15019,#15020);
#13979=AXIS2_PLACEMENT_3D('',#18394,#15021,#15022);
#13980=AXIS2_PLACEMENT_3D('',#18400,#15026,#15027);
#13981=AXIS2_PLACEMENT_3D('',#18404,#15029,#15030);
#13982=AXIS2_PLACEMENT_3D('',#18405,#15031,#15032);
#13983=AXIS2_PLACEMENT_3D('',#18406,#15033,#15034);
#13984=AXIS2_PLACEMENT_3D('',#18412,#15038,#15039);
#13985=AXIS2_PLACEMENT_3D('',#18416,#15041,#15042);
#13986=AXIS2_PLACEMENT_3D('',#18417,#15043,#15044);
#13987=AXIS2_PLACEMENT_3D('',#18418,#15045,#15046);
#13988=AXIS2_PLACEMENT_3D('',#18424,#15050,#15051);
#13989=AXIS2_PLACEMENT_3D('',#18425,#15052,#15053);
#13990=AXIS2_PLACEMENT_3D('',#18426,#15054,#15055);
#13991=AXIS2_PLACEMENT_3D('',#18427,#15056,#15057);
#13992=AXIS2_PLACEMENT_3D('',#18431,#15059,#15060);
#13993=AXIS2_PLACEMENT_3D('',#18433,#15062,#15063);
#13994=AXIS2_PLACEMENT_3D('',#18438,#15066,#15067);
#13995=AXIS2_PLACEMENT_3D('',#18439,#15068,#15069);
#13996=AXIS2_PLACEMENT_3D('',#18442,#15071,#15072);
#13997=AXIS2_PLACEMENT_3D('',#18443,#15073,#15074);
#13998=AXIS2_PLACEMENT_3D('',#18447,#15077,#15078);
#13999=AXIS2_PLACEMENT_3D('',#18452,#15080,#15081);
#14000=AXIS2_PLACEMENT_3D('',#18456,#15083,#15084);
#14001=AXIS2_PLACEMENT_3D('',#18460,#15086,#15087);
#14002=AXIS2_PLACEMENT_3D('',#18463,#15089,#15090);
#14003=AXIS2_PLACEMENT_3D('',#18464,#15091,#15092);
#14004=AXIS2_PLACEMENT_3D('',#18470,#15096,#15097);
#14005=AXIS2_PLACEMENT_3D('',#18473,#15099,#15100);
#14006=AXIS2_PLACEMENT_3D('',#18474,#15101,#15102);
#14007=AXIS2_PLACEMENT_3D('',#18478,#15105,#15106);
#14008=AXIS2_PLACEMENT_3D('',#18481,#15108,#15109);
#14009=AXIS2_PLACEMENT_3D('',#18482,#15110,#15111);
#14010=AXIS2_PLACEMENT_3D('',#18486,#15114,#15115);
#14011=AXIS2_PLACEMENT_3D('',#18489,#15117,#15118);
#14012=AXIS2_PLACEMENT_3D('',#18490,#15119,#15120);
#14013=AXIS2_PLACEMENT_3D('',#18494,#15123,#15124);
#14014=AXIS2_PLACEMENT_3D('',#18495,#15125,#15126);
#14015=AXIS2_PLACEMENT_3D('',#18496,#15127,#15128);
#14016=AXIS2_PLACEMENT_3D('',#18500,#15130,#15131);
#14017=AXIS2_PLACEMENT_3D('',#18502,#15133,#15134);
#14018=AXIS2_PLACEMENT_3D('',#18506,#15137,#15138);
#14019=AXIS2_PLACEMENT_3D('',#18509,#15140,#15141);
#14020=AXIS2_PLACEMENT_3D('',#18510,#15142,#15143);
#14021=AXIS2_PLACEMENT_3D('',#18514,#15146,#15147);
#14022=AXIS2_PLACEMENT_3D('',#18520,#15151,#15152);
#14023=AXIS2_PLACEMENT_3D('',#18523,#15154,#15155);
#14024=AXIS2_PLACEMENT_3D('',#18524,#15156,#15157);
#14025=AXIS2_PLACEMENT_3D('',#18530,#15161,#15162);
#14026=AXIS2_PLACEMENT_3D('',#18534,#15164,#15165);
#14027=AXIS2_PLACEMENT_3D('',#18535,#15166,#15167);
#14028=AXIS2_PLACEMENT_3D('',#18536,#15168,#15169);
#14029=AXIS2_PLACEMENT_3D('',#18542,#15173,#15174);
#14030=AXIS2_PLACEMENT_3D('',#18545,#15176,#15177);
#14031=AXIS2_PLACEMENT_3D('',#18546,#15178,#15179);
#14032=AXIS2_PLACEMENT_3D('',#18547,#15180,#15181);
#14033=AXIS2_PLACEMENT_3D('',#18551,#15184,#15185);
#14034=AXIS2_PLACEMENT_3D('',#18552,#15186,#15187);
#14035=AXIS2_PLACEMENT_3D('',#18553,#15188,#15189);
#14036=AXIS2_PLACEMENT_3D('',#18555,#15191,#15192);
#14037=AXIS2_PLACEMENT_3D('',#18560,#15194,#15195);
#14038=AXIS2_PLACEMENT_3D('',#18564,#15197,#15198);
#14039=AXIS2_PLACEMENT_3D('',#18568,#15200,#15201);
#14040=AXIS2_PLACEMENT_3D('',#18571,#15203,#15204);
#14041=AXIS2_PLACEMENT_3D('',#18572,#15205,#15206);
#14042=AXIS2_PLACEMENT_3D('',#18575,#15209,#15210);
#14043=AXIS2_PLACEMENT_3D('',#18577,#15212,#15213);
#14044=AXIS2_PLACEMENT_3D('',#18581,#15216,#15217);
#14045=AXIS2_PLACEMENT_3D('',#18584,#15219,#15220);
#14046=AXIS2_PLACEMENT_3D('',#18585,#15221,#15222);
#14047=AXIS2_PLACEMENT_3D('',#18589,#15225,#15226);
#14048=AXIS2_PLACEMENT_3D('',#18591,#15228,#15229);
#14049=AXIS2_PLACEMENT_3D('',#18592,#15230,#15231);
#14050=AXIS2_PLACEMENT_3D('',#18594,#15233,#15234);
#14051=AXIS2_PLACEMENT_3D('',#18595,#15235,#15236);
#14052=AXIS2_PLACEMENT_3D('',#18597,#15238,#15239);
#14053=AXIS2_PLACEMENT_3D('',#18599,#15240,#15241);
#14054=AXIS2_PLACEMENT_3D('',#18601,#15243,#15244);
#14055=AXIS2_PLACEMENT_3D('',#18603,#15246,#15247);
#14056=AXIS2_PLACEMENT_3D('',#18605,#15249,#15250);
#14057=AXIS2_PLACEMENT_3D('',#18606,#15251,#15252);
#14058=AXIS2_PLACEMENT_3D('',#18608,#15254,#15255);
#14059=AXIS2_PLACEMENT_3D('',#18610,#15257,#15258);
#15006=DIRECTION('axis',(0.,0.,1.));
#15007=DIRECTION('refdir',(1.,0.,0.));
#15008=DIRECTION('center_axis',(0.707106781186541,-0.707106781186554,0.));
#15009=DIRECTION('ref_axis',(0.,0.,-1.));
#15010=DIRECTION('',(0.707106781186554,0.707106781186541,-6.28036983473507E-15));
#15011=DIRECTION('',(0.,0.,1.));
#15012=DIRECTION('',(-0.707106781186554,-0.707106781186541,0.));
#15013=DIRECTION('',(0.,0.,-1.));
#15014=DIRECTION('center_axis',(1.,0.,0.));
#15015=DIRECTION('ref_axis',(0.,-3.96951249027992E-15,-1.));
#15016=DIRECTION('',(0.707106781186554,0.,-0.707106781186541));
#15017=DIRECTION('center_axis',(1.,0.,0.));
#15018=DIRECTION('ref_axis',(0.,-3.96951249027992E-15,-1.));
#15019=DIRECTION('center_axis',(-1.,0.,0.));
#15020=DIRECTION('ref_axis',(0.,-3.96951249027992E-15,-1.));
#15021=DIRECTION('center_axis',(0.707106781186541,0.,0.707106781186554));
#15022=DIRECTION('ref_axis',(0.707106781186554,0.,-0.707106781186541));
#15023=DIRECTION('',(0.707106781186554,3.14018491736753E-15,-0.707106781186541));
#15024=DIRECTION('',(0.,1.,0.));
#15025=DIRECTION('',(0.,-1.,0.));
#15026=DIRECTION('center_axis',(1.,0.,0.));
#15027=DIRECTION('ref_axis',(0.,-1.,-1.98475624513994E-15));
#15028=DIRECTION('',(0.707106781186553,-0.707106781186542,0.));
#15029=DIRECTION('center_axis',(1.,0.,0.));
#15030=DIRECTION('ref_axis',(0.,-1.,-1.98475624513994E-15));
#15031=DIRECTION('center_axis',(-1.,0.,0.));
#15032=DIRECTION('ref_axis',(0.,-1.,-1.98475624513994E-15));
#15033=DIRECTION('center_axis',(0.707106781186542,0.707106781186553,0.));
#15034=DIRECTION('ref_axis',(0.,0.,-1.));
#15035=DIRECTION('',(0.707106781186554,-0.707106781186541,0.));
#15036=DIRECTION('',(0.,0.,-1.));
#15037=DIRECTION('',(0.,0.,1.));
#15038=DIRECTION('center_axis',(1.,0.,0.));
#15039=DIRECTION('ref_axis',(0.,-9.92378122569971E-16,1.));
#15040=DIRECTION('',(0.707106781186554,0.,0.707106781186541));
#15041=DIRECTION('center_axis',(1.,0.,0.));
#15042=DIRECTION('ref_axis',(0.,-9.92378122569971E-16,1.));
#15043=DIRECTION('center_axis',(-1.,0.,0.));
#15044=DIRECTION('ref_axis',(0.,-9.92378122569971E-16,1.));
#15045=DIRECTION('center_axis',(0.707106781186541,0.,-0.707106781186554));
#15046=DIRECTION('ref_axis',(-0.707106781186554,0.,-0.707106781186541));
#15047=DIRECTION('',(0.707106781186551,0.,0.707106781186544));
#15048=DIRECTION('',(0.,-1.,0.));
#15049=DIRECTION('',(0.,1.,0.));
#15050=DIRECTION('center_axis',(1.,0.,0.));
#15051=DIRECTION('ref_axis',(0.,1.,-5.95426873541988E-15));
#15052=DIRECTION('center_axis',(1.,0.,0.));
#15053=DIRECTION('ref_axis',(0.,1.,-5.95426873541988E-15));
#15054=DIRECTION('center_axis',(-1.,0.,0.));
#15055=DIRECTION('ref_axis',(0.,1.,-5.95426873541988E-15));
#15056=DIRECTION('center_axis',(1.,0.,0.));
#15057=DIRECTION('ref_axis',(0.,-1.,-1.98475624513994E-15));
#15058=DIRECTION('',(1.,0.,0.));
#15059=DIRECTION('center_axis',(1.,0.,0.));
#15060=DIRECTION('ref_axis',(0.,-1.,-1.98475624513994E-15));
#15061=DIRECTION('',(1.,0.,0.));
#15062=DIRECTION('center_axis',(0.,0.,1.));
#15063=DIRECTION('ref_axis',(0.,-1.,0.));
#15064=DIRECTION('',(1.,0.,0.));
#15065=DIRECTION('',(0.,1.,0.));
#15066=DIRECTION('center_axis',(0.,0.,-1.));
#15067=DIRECTION('ref_axis',(1.,0.,0.));
#15068=DIRECTION('center_axis',(1.,0.,0.));
#15069=DIRECTION('ref_axis',(0.,-3.96951249027992E-15,-1.));
#15070=DIRECTION('',(1.,0.,0.));
#15071=DIRECTION('center_axis',(1.,0.,0.));
#15072=DIRECTION('ref_axis',(0.,-3.96951249027992E-15,-1.));
#15073=DIRECTION('center_axis',(0.,-1.,0.));
#15074=DIRECTION('ref_axis',(0.,0.,-1.));
#15075=DIRECTION('',(1.,0.,0.));
#15076=DIRECTION('',(0.,0.,1.));
#15077=DIRECTION('center_axis',(1.,0.,0.));
#15078=DIRECTION('ref_axis',(0.,0.,-1.));
#15079=DIRECTION('',(0.,1.,0.));
#15080=DIRECTION('center_axis',(-1.,0.,0.));
#15081=DIRECTION('ref_axis',(0.,4.75809867696496E-16,1.));
#15082=DIRECTION('',(0.,0.,1.));
#15083=DIRECTION('center_axis',(-1.,0.,0.));
#15084=DIRECTION('ref_axis',(0.,-1.,0.));
#15085=DIRECTION('',(0.,-1.,0.));
#15086=DIRECTION('center_axis',(-1.,0.,0.));
#15087=DIRECTION('ref_axis',(0.,1.26882631385732E-15,-1.));
#15088=DIRECTION('',(0.,0.,-1.));
#15089=DIRECTION('center_axis',(-1.,0.,0.));
#15090=DIRECTION('ref_axis',(0.,1.,6.34413156928661E-16));
#15091=DIRECTION('center_axis',(0.707106781186541,0.,0.707106781186554));
#15092=DIRECTION('ref_axis',(0.707106781186554,0.,-0.707106781186541));
#15093=DIRECTION('',(0.707106781186554,3.14018491736753E-15,-0.707106781186541));
#15094=DIRECTION('',(-0.707106781186554,0.,0.707106781186541));
#15095=DIRECTION('',(0.,-1.,0.));
#15096=DIRECTION('center_axis',(-1.,0.,0.));
#15097=DIRECTION('ref_axis',(0.,4.75809867696496E-16,1.));
#15098=DIRECTION('',(0.707106781186553,0.707106781186542,0.));
#15099=DIRECTION('center_axis',(1.,0.,0.));
#15100=DIRECTION('ref_axis',(0.,4.75809867696496E-16,1.));
#15101=DIRECTION('center_axis',(0.707106781186543,-0.707106781186552,0.));
#15102=DIRECTION('ref_axis',(0.,0.,-1.));
#15103=DIRECTION('',(0.707106781186552,0.707106781186543,-6.28036983473505E-15));
#15104=DIRECTION('',(0.,0.,-1.));
#15105=DIRECTION('center_axis',(-1.,0.,0.));
#15106=DIRECTION('ref_axis',(0.,-1.,0.));
#15107=DIRECTION('',(0.707106781186554,0.,0.707106781186541));
#15108=DIRECTION('center_axis',(1.,0.,0.));
#15109=DIRECTION('ref_axis',(0.,-1.,0.));
#15110=DIRECTION('center_axis',(0.707106781186541,0.,-0.707106781186554));
#15111=DIRECTION('ref_axis',(-0.707106781186554,0.,-0.707106781186541));
#15112=DIRECTION('',(0.707106781186554,0.,0.707106781186541));
#15113=DIRECTION('',(0.,1.,0.));
#15114=DIRECTION('center_axis',(-1.,0.,0.));
#15115=DIRECTION('ref_axis',(0.,1.26882631385732E-15,-1.));
#15116=DIRECTION('',(0.70710678118656,-0.707106781186535,0.));
#15117=DIRECTION('center_axis',(1.,0.,0.));
#15118=DIRECTION('ref_axis',(0.,1.26882631385732E-15,-1.));
#15119=DIRECTION('center_axis',(0.707106781186541,0.707106781186554,0.));
#15120=DIRECTION('ref_axis',(0.,0.,-1.));
#15121=DIRECTION('',(0.707106781186554,-0.707106781186541,6.28036983473507E-15));
#15122=DIRECTION('',(0.,0.,1.));
#15123=DIRECTION('center_axis',(-1.,0.,0.));
#15124=DIRECTION('ref_axis',(0.,1.,6.34413156928661E-16));
#15125=DIRECTION('center_axis',(1.,0.,0.));
#15126=DIRECTION('ref_axis',(0.,1.,6.34413156928661E-16));
#15127=DIRECTION('center_axis',(1.,0.,0.));
#15128=DIRECTION('ref_axis',(0.,-1.,0.));
#15129=DIRECTION('',(1.,0.,0.));
#15130=DIRECTION('center_axis',(-1.,0.,0.));
#15131=DIRECTION('ref_axis',(0.,-1.,0.));
#15132=DIRECTION('',(1.,0.,0.));
#15133=DIRECTION('center_axis',(0.,-1.,0.));
#15134=DIRECTION('ref_axis',(0.,0.,-1.));
#15135=DIRECTION('',(1.,0.,0.));
#15136=DIRECTION('',(0.,0.,1.));
#15137=DIRECTION('center_axis',(1.,0.,0.));
#15138=DIRECTION('ref_axis',(0.,4.75809867696496E-16,1.));
#15139=DIRECTION('',(1.,0.,0.));
#15140=DIRECTION('center_axis',(-1.,0.,0.));
#15141=DIRECTION('ref_axis',(0.,4.75809867696496E-16,1.));
#15142=DIRECTION('center_axis',(0.,0.,1.));
#15143=DIRECTION('ref_axis',(0.,-1.,0.));
#15144=DIRECTION('',(1.,0.,0.));
#15145=DIRECTION('',(0.,1.,0.));
#15146=DIRECTION('center_axis',(-0.707106781186548,-0.707106781186547,0.));
#15147=DIRECTION('ref_axis',(0.,0.,1.));
#15148=DIRECTION('',(0.707106781186547,-0.707106781186548,5.23364152894591E-15));
#15149=DIRECTION('',(-0.707106781186547,0.707106781186548,0.));
#15150=DIRECTION('',(0.,0.,-1.));
#15151=DIRECTION('center_axis',(1.,0.,0.));
#15152=DIRECTION('ref_axis',(0.,-1.,0.));
#15153=DIRECTION('',(0.707106781186547,0.,-0.707106781186548));
#15154=DIRECTION('center_axis',(1.,0.,0.));
#15155=DIRECTION('ref_axis',(0.,-1.,0.));
#15156=DIRECTION('center_axis',(-0.707106781186548,0.,-0.707106781186547));
#15157=DIRECTION('ref_axis',(-0.707106781186547,0.,0.707106781186548));
#15158=DIRECTION('',(0.707106781186547,0.,-0.707106781186548));
#15159=DIRECTION('',(0.,-1.,0.));
#15160=DIRECTION('',(0.,1.,0.));
#15161=DIRECTION('center_axis',(1.,0.,0.));
#15162=DIRECTION('ref_axis',(0.,1.26882631385732E-15,-1.));
#15163=DIRECTION('',(0.707106781186555,0.70710678118654,0.));
#15164=DIRECTION('center_axis',(-1.,0.,0.));
#15165=DIRECTION('ref_axis',(0.,1.26882631385732E-15,-1.));
#15166=DIRECTION('center_axis',(1.,0.,0.));
#15167=DIRECTION('ref_axis',(0.,1.26882631385732E-15,-1.));
#15168=DIRECTION('center_axis',(-0.707106781186545,0.70710678118655,0.));
#15169=DIRECTION('ref_axis',(0.,0.,1.));
#15170=DIRECTION('',(0.70710678118655,0.707106781186545,-5.23364152894593E-15));
#15171=DIRECTION('',(0.,0.,-1.));
#15172=DIRECTION('',(0.,0.,1.));
#15173=DIRECTION('center_axis',(1.,0.,0.));
#15174=DIRECTION('ref_axis',(0.,1.,6.34413156928661E-16));
#15175=DIRECTION('',(0.70710678118655,0.,0.707106781186545));
#15176=DIRECTION('center_axis',(-1.,0.,0.));
#15177=DIRECTION('ref_axis',(0.,1.,6.34413156928661E-16));
#15178=DIRECTION('center_axis',(1.,0.,0.));
#15179=DIRECTION('ref_axis',(0.,1.,6.34413156928661E-16));
#15180=DIRECTION('center_axis',(-0.707106781186548,0.,0.707106781186547));
#15181=DIRECTION('ref_axis',(0.707106781186547,0.,0.707106781186548));
#15182=DIRECTION('',(0.707106781186547,-2.61682076447296E-15,0.707106781186548));
#15183=DIRECTION('',(0.,-1.,0.));
#15184=DIRECTION('center_axis',(1.,0.,0.));
#15185=DIRECTION('ref_axis',(0.,4.75809867696496E-16,1.));
#15186=DIRECTION('center_axis',(1.,0.,0.));
#15187=DIRECTION('ref_axis',(0.,4.75809867696496E-16,1.));
#15188=DIRECTION('center_axis',(1.,0.,0.));
#15189=DIRECTION('ref_axis',(0.,1.,6.34413156928661E-16));
#15190=DIRECTION('',(1.,0.,0.));
#15191=DIRECTION('center_axis',(1.,0.,0.));
#15192=DIRECTION('ref_axis',(0.,0.,-1.));
#15193=DIRECTION('',(0.,-1.,0.));
#15194=DIRECTION('center_axis',(-1.,0.,0.));
#15195=DIRECTION('ref_axis',(0.,-3.96951249027992E-15,-1.));
#15196=DIRECTION('',(0.,0.,-1.));
#15197=DIRECTION('center_axis',(-1.,0.,0.));
#15198=DIRECTION('ref_axis',(0.,1.,-5.95426873541988E-15));
#15199=DIRECTION('',(0.,1.,0.));
#15200=DIRECTION('center_axis',(-1.,0.,0.));
#15201=DIRECTION('ref_axis',(0.,-9.92378122569971E-16,1.));
#15202=DIRECTION('',(0.,0.,1.));
#15203=DIRECTION('center_axis',(-1.,0.,0.));
#15204=DIRECTION('ref_axis',(0.,-1.,-1.98475624513994E-15));
#15205=DIRECTION('center_axis',(-0.707106781186548,0.,0.707106781186547));
#15206=DIRECTION('ref_axis',(0.707106781186547,0.,0.707106781186548));
#15207=DIRECTION('',(0.707106781186547,-2.61682076447296E-15,0.707106781186548));
#15208=DIRECTION('',(-0.707106781186547,0.,-0.707106781186548));
#15209=DIRECTION('center_axis',(-1.,0.,0.));
#15210=DIRECTION('ref_axis',(0.,-1.,-1.98475624513994E-15));
#15211=DIRECTION('',(0.707106781186547,0.707106781186548,0.));
#15212=DIRECTION('center_axis',(-0.707106781186548,0.707106781186547,0.));
#15213=DIRECTION('ref_axis',(0.,0.,1.));
#15214=DIRECTION('',(0.707106781186547,0.707106781186548,0.));
#15215=DIRECTION('',(0.,0.,-1.));
#15216=DIRECTION('center_axis',(-1.,0.,0.));
#15217=DIRECTION('ref_axis',(0.,-9.92378122569971E-16,1.));
#15218=DIRECTION('',(0.707106781186547,1.30841038223648E-15,-0.707106781186548));
#15219=DIRECTION('center_axis',(1.,0.,0.));
#15220=DIRECTION('ref_axis',(0.,-9.92378122569971E-16,1.));
#15221=DIRECTION('center_axis',(-0.707106781186548,0.,-0.707106781186547));
#15222=DIRECTION('ref_axis',(-0.707106781186547,0.,0.707106781186548));
#15223=DIRECTION('',(0.707106781186545,0.,-0.70710678118655));
#15224=DIRECTION('',(0.,-1.,0.));
#15225=DIRECTION('center_axis',(-1.,0.,0.));
#15226=DIRECTION('ref_axis',(0.,1.,-5.95426873541988E-15));
#15227=DIRECTION('',(0.70710678118655,-0.707106781186545,5.23364152894593E-15));
#15228=DIRECTION('center_axis',(1.,0.,0.));
#15229=DIRECTION('ref_axis',(0.,1.,-5.95426873541988E-15));
#15230=DIRECTION('center_axis',(-0.707106781186545,-0.70710678118655,0.));
#15231=DIRECTION('ref_axis',(0.,0.,1.));
#15232=DIRECTION('',(0.70710678118655,-0.707106781186545,5.23364152894593E-15));
#15233=DIRECTION('center_axis',(-1.,0.,0.));
#15234=DIRECTION('ref_axis',(0.,-3.96951249027992E-15,-1.));
#15235=DIRECTION('center_axis',(1.,0.,0.));
#15236=DIRECTION('ref_axis',(0.,1.,-5.95426873541988E-15));
#15237=DIRECTION('',(1.,0.,0.));
#15238=DIRECTION('center_axis',(0.,0.,1.));
#15239=DIRECTION('ref_axis',(1.,0.,0.));
#15240=DIRECTION('center_axis',(0.,0.,1.));
#15241=DIRECTION('ref_axis',(1.,0.,0.));
#15242=DIRECTION('',(0.,0.,1.));
#15243=DIRECTION('center_axis',(0.,0.,-1.));
#15244=DIRECTION('ref_axis',(0.,1.,0.));
#15245=DIRECTION('',(1.,0.,0.));
#15246=DIRECTION('center_axis',(1.,0.,0.));
#15247=DIRECTION('ref_axis',(0.,-9.92378122569971E-16,1.));
#15248=DIRECTION('',(1.,0.,0.));
#15249=DIRECTION('center_axis',(0.,1.,0.));
#15250=DIRECTION('ref_axis',(0.,0.,1.));
#15251=DIRECTION('center_axis',(0.,1.,0.));
#15252=DIRECTION('ref_axis',(0.,0.,1.));
#15253=DIRECTION('',(1.,0.,0.));
#15254=DIRECTION('center_axis',(1.,0.,0.));
#15255=DIRECTION('ref_axis',(0.,1.26882631385732E-15,-1.));
#15256=DIRECTION('',(1.,0.,0.));
#15257=DIRECTION('center_axis',(0.,0.,-1.));
#15258=DIRECTION('ref_axis',(0.,1.,0.));
#18378=CARTESIAN_POINT('',(0.,0.,0.));
#18379=CARTESIAN_POINT('Origin',(177.55,58.9875,12.375));
#18380=CARTESIAN_POINT('',(177.3,58.7375,-24.75));
#18381=CARTESIAN_POINT('',(177.8,59.2375,-24.75));
#18382=CARTESIAN_POINT('',(177.3,58.7375,-24.75));
#18383=CARTESIAN_POINT('',(177.8,59.2375,24.75));
#18384=CARTESIAN_POINT('',(177.8,59.2375,12.375));
#18385=CARTESIAN_POINT('',(177.3,58.7375,24.75));
#18386=CARTESIAN_POINT('',(177.8,59.2375,24.75));
#18387=CARTESIAN_POINT('',(177.3,58.7375,12.375));
#18388=CARTESIAN_POINT('Origin',(177.55,56.5,-24.75));
#18389=CARTESIAN_POINT('',(177.3,56.5,-26.9875));
#18390=CARTESIAN_POINT('',(177.8,56.5,-27.4875));
#18391=CARTESIAN_POINT('',(177.3,56.5,-26.9875));
#18392=CARTESIAN_POINT('Origin',(177.8,56.5,-24.75));
#18393=CARTESIAN_POINT('Origin',(177.3,56.5,-24.75));
#18394=CARTESIAN_POINT('Origin',(177.55,44.125,-27.2375));
#18395=CARTESIAN_POINT('',(177.3,7.,-26.9875));
#18396=CARTESIAN_POINT('',(177.8,7.,-27.4875));
#18397=CARTESIAN_POINT('',(177.3,7.,-26.9875));
#18398=CARTESIAN_POINT('',(177.8,44.125,-27.4875));
#18399=CARTESIAN_POINT('',(177.3,44.125,-26.9875));
#18400=CARTESIAN_POINT('Origin',(177.55,7.,-24.75));
#18401=CARTESIAN_POINT('',(177.3,4.7625,-24.75));
#18402=CARTESIAN_POINT('',(177.8,4.2625,-24.75));
#18403=CARTESIAN_POINT('',(177.3,4.7625,-24.75));
#18404=CARTESIAN_POINT('Origin',(177.8,7.,-24.75));
#18405=CARTESIAN_POINT('Origin',(177.3,7.,-24.75));
#18406=CARTESIAN_POINT('Origin',(177.55,4.5125,-12.375));
#18407=CARTESIAN_POINT('',(177.3,4.7625,24.75));
#18408=CARTESIAN_POINT('',(177.8,4.2625,24.75));
#18409=CARTESIAN_POINT('',(177.3,4.7625,24.75));
#18410=CARTESIAN_POINT('',(177.8,4.2625,-12.375));
#18411=CARTESIAN_POINT('',(177.3,4.7625,-12.375));
#18412=CARTESIAN_POINT('Origin',(177.55,7.,24.75));
#18413=CARTESIAN_POINT('',(177.3,7.,26.9875));
#18414=CARTESIAN_POINT('',(177.8,7.,27.4875));
#18415=CARTESIAN_POINT('',(177.3,7.,26.9875));
#18416=CARTESIAN_POINT('Origin',(177.8,7.,24.75));
#18417=CARTESIAN_POINT('Origin',(177.3,7.,24.75));
#18418=CARTESIAN_POINT('Origin',(177.55,19.375,27.2375));
#18419=CARTESIAN_POINT('',(177.3,56.5,26.9875));
#18420=CARTESIAN_POINT('',(177.8,56.5,27.4875));
#18421=CARTESIAN_POINT('',(177.3,56.5,26.9875));
#18422=CARTESIAN_POINT('',(177.8,19.375,27.4875));
#18423=CARTESIAN_POINT('',(177.3,19.375,26.9875));
#18424=CARTESIAN_POINT('Origin',(177.55,56.5,24.75));
#18425=CARTESIAN_POINT('Origin',(177.8,56.5,24.75));
#18426=CARTESIAN_POINT('Origin',(177.3,56.5,24.75));
#18427=CARTESIAN_POINT('Origin',(0.,7.,-24.75));
#18428=CARTESIAN_POINT('',(0.6,7.,-26.9875));
#18429=CARTESIAN_POINT('',(0.,7.,-26.9875));
#18430=CARTESIAN_POINT('',(0.6,4.7625,-24.75));
#18431=CARTESIAN_POINT('Origin',(0.6,7.,-24.75));
#18432=CARTESIAN_POINT('',(0.,4.7625,-24.75));
#18433=CARTESIAN_POINT('Origin',(0.,56.5,-26.9875));
#18434=CARTESIAN_POINT('',(0.6,56.5,-26.9875));
#18435=CARTESIAN_POINT('',(0.,56.5,-26.9875));
#18436=CARTESIAN_POINT('',(0.6,44.125,-26.9875));
#18437=CARTESIAN_POINT('',(10.,31.75,-26.9875));
#18438=CARTESIAN_POINT('Origin',(15.2,31.75,-26.9875));
#18439=CARTESIAN_POINT('Origin',(0.,56.5,-24.75));
#18440=CARTESIAN_POINT('',(0.6,58.7375,-24.75));
#18441=CARTESIAN_POINT('',(0.,58.7375,-24.75));
#18442=CARTESIAN_POINT('Origin',(0.6,56.5,-24.75));
#18443=CARTESIAN_POINT('Origin',(0.,58.7375,24.75));
#18444=CARTESIAN_POINT('',(0.6,58.7375,24.75));
#18445=CARTESIAN_POINT('',(0.,58.7375,24.75));
#18446=CARTESIAN_POINT('',(0.6,58.7375,12.375));
#18447=CARTESIAN_POINT('Origin',(177.8,31.75,0.));
#18448=CARTESIAN_POINT('',(177.8,7.,31.25));
#18449=CARTESIAN_POINT('',(177.8,56.5,31.25));
#18450=CARTESIAN_POINT('',(177.8,44.125,31.25));
#18451=CARTESIAN_POINT('',(177.8,0.499999999999998,24.75));
#18452=CARTESIAN_POINT('Origin',(177.8,7.,24.75));
#18453=CARTESIAN_POINT('',(177.8,0.5,-24.75));
#18454=CARTESIAN_POINT('',(177.8,0.5,12.375));
#18455=CARTESIAN_POINT('',(177.8,7.,-31.25));
#18456=CARTESIAN_POINT('Origin',(177.8,7.,-24.75));
#18457=CARTESIAN_POINT('',(177.8,56.5,-31.25));
#18458=CARTESIAN_POINT('',(177.8,19.375,-31.25));
#18459=CARTESIAN_POINT('',(177.8,63.,-24.75));
#18460=CARTESIAN_POINT('Origin',(177.8,56.5,-24.75));
#18461=CARTESIAN_POINT('',(177.8,63.,24.75));
#18462=CARTESIAN_POINT('',(177.8,63.,-12.375));
#18463=CARTESIAN_POINT('Origin',(177.8,56.5,24.75));
#18464=CARTESIAN_POINT('Origin',(177.55,44.125,31.5));
#18465=CARTESIAN_POINT('',(177.3,7.,31.75));
#18466=CARTESIAN_POINT('',(177.3,7.,31.75));
#18467=CARTESIAN_POINT('',(177.3,56.5,31.75));
#18468=CARTESIAN_POINT('',(177.8,56.5,31.25));
#18469=CARTESIAN_POINT('',(177.3,44.125,31.75));
#18470=CARTESIAN_POINT('Origin',(177.55,7.,24.75));
#18471=CARTESIAN_POINT('',(177.3,-1.11022302462516E-15,24.75));
#18472=CARTESIAN_POINT('',(177.3,-1.11022302462516E-15,24.75));
#18473=CARTESIAN_POINT('Origin',(177.3,7.,24.75));
#18474=CARTESIAN_POINT('Origin',(177.55,0.25,12.375));
#18475=CARTESIAN_POINT('',(177.3,0.,-24.75));
#18476=CARTESIAN_POINT('',(177.3,0.,-24.75));
#18477=CARTESIAN_POINT('',(177.3,0.,12.375));
#18478=CARTESIAN_POINT('Origin',(177.55,7.,-24.75));
#18479=CARTESIAN_POINT('',(177.3,7.,-31.75));
#18480=CARTESIAN_POINT('',(177.3,7.,-31.75));
#18481=CARTESIAN_POINT('Origin',(177.3,7.,-24.75));
#18482=CARTESIAN_POINT('Origin',(177.55,19.375,-31.5));
#18483=CARTESIAN_POINT('',(177.3,56.5,-31.75));
#18484=CARTESIAN_POINT('',(177.3,56.5,-31.75));
#18485=CARTESIAN_POINT('',(177.3,19.375,-31.75));
#18486=CARTESIAN_POINT('Origin',(177.55,56.5,-24.75));
#18487=CARTESIAN_POINT('',(177.3,63.5,-24.75));
#18488=CARTESIAN_POINT('',(177.3,63.5,-24.75));
#18489=CARTESIAN_POINT('Origin',(177.3,56.5,-24.75));
#18490=CARTESIAN_POINT('Origin',(177.55,63.25,-12.375));
#18491=CARTESIAN_POINT('',(177.3,63.5,24.75));
#18492=CARTESIAN_POINT('',(177.3,63.5,24.75));
#18493=CARTESIAN_POINT('',(177.3,63.5,-12.375));
#18494=CARTESIAN_POINT('Origin',(177.55,56.5,24.75));
#18495=CARTESIAN_POINT('Origin',(177.3,56.5,24.75));
#18496=CARTESIAN_POINT('Origin',(0.,7.,-24.75));
#18497=CARTESIAN_POINT('',(0.6,0.,-24.75));
#18498=CARTESIAN_POINT('',(0.,0.,-24.75));
#18499=CARTESIAN_POINT('',(0.6,7.,-31.75));
#18500=CARTESIAN_POINT('Origin',(0.6,7.,-24.75));
#18501=CARTESIAN_POINT('',(0.,7.,-31.75));
#18502=CARTESIAN_POINT('Origin',(0.,0.,24.75));
#18503=CARTESIAN_POINT('',(0.6,-1.11022302462516E-15,24.75));
#18504=CARTESIAN_POINT('',(0.,-1.11022302462516E-15,24.75));
#18505=CARTESIAN_POINT('',(0.6,0.,12.375));
#18506=CARTESIAN_POINT('Origin',(0.,7.,24.75));
#18507=CARTESIAN_POINT('',(0.6,7.,31.75));
#18508=CARTESIAN_POINT('',(0.,7.,31.75));
#18509=CARTESIAN_POINT('Origin',(0.6,7.,24.75));
#18510=CARTESIAN_POINT('Origin',(0.,56.5,31.75));
#18511=CARTESIAN_POINT('',(0.6,56.5,31.75));
#18512=CARTESIAN_POINT('',(0.,56.5,31.75));
#18513=CARTESIAN_POINT('',(0.6,44.125,31.75));
#18514=CARTESIAN_POINT('Origin',(0.3,0.3,12.375));
#18515=CARTESIAN_POINT('',(0.,0.600000000000001,-24.75));
#18516=CARTESIAN_POINT('',(0.,0.600000000000001,-24.75));
#18517=CARTESIAN_POINT('',(0.,0.600000000000001,24.75));
#18518=CARTESIAN_POINT('',(0.6,-1.11022302462516E-15,24.75));
#18519=CARTESIAN_POINT('',(0.,0.600000000000001,12.375));
#18520=CARTESIAN_POINT('Origin',(0.3,7.,-24.75));
#18521=CARTESIAN_POINT('',(0.,7.,-31.15));
#18522=CARTESIAN_POINT('',(0.,7.,-31.15));
#18523=CARTESIAN_POINT('Origin',(0.,7.,-24.75));
#18524=CARTESIAN_POINT('Origin',(0.3,19.375,-31.45));
#18525=CARTESIAN_POINT('',(0.,56.5,-31.15));
#18526=CARTESIAN_POINT('',(0.6,56.5,-31.75));
#18527=CARTESIAN_POINT('',(0.,56.5,-31.15));
#18528=CARTESIAN_POINT('',(0.6,19.375,-31.75));
#18529=CARTESIAN_POINT('',(0.,19.375,-31.15));
#18530=CARTESIAN_POINT('Origin',(0.3,56.5,-24.75));
#18531=CARTESIAN_POINT('',(0.,62.9,-24.75));
#18532=CARTESIAN_POINT('',(0.6,63.5,-24.75));
#18533=CARTESIAN_POINT('',(0.,62.9,-24.75));
#18534=CARTESIAN_POINT('Origin',(0.6,56.5,-24.75));
#18535=CARTESIAN_POINT('Origin',(0.,56.5,-24.75));
#18536=CARTESIAN_POINT('Origin',(0.3,63.2,-12.375));
#18537=CARTESIAN_POINT('',(0.,62.9,24.75));
#18538=CARTESIAN_POINT('',(0.6,63.5,24.75));
#18539=CARTESIAN_POINT('',(0.,62.9,24.75));
#18540=CARTESIAN_POINT('',(0.6,63.5,-12.375));
#18541=CARTESIAN_POINT('',(0.,62.9,-12.375));
#18542=CARTESIAN_POINT('Origin',(0.3,56.5,24.75));
#18543=CARTESIAN_POINT('',(0.,56.5,31.15));
#18544=CARTESIAN_POINT('',(0.,56.5,31.15));
#18545=CARTESIAN_POINT('Origin',(0.6,56.5,24.75));
#18546=CARTESIAN_POINT('Origin',(0.,56.5,24.75));
#18547=CARTESIAN_POINT('Origin',(0.3,44.125,31.45));
#18548=CARTESIAN_POINT('',(0.,7.,31.15));
#18549=CARTESIAN_POINT('',(0.,7.,31.15));
#18550=CARTESIAN_POINT('',(0.,44.125,31.15));
#18551=CARTESIAN_POINT('Origin',(0.3,7.,24.75));
#18552=CARTESIAN_POINT('Origin',(0.,7.,24.75));
#18553=CARTESIAN_POINT('Origin',(0.,56.5,24.75));
#18554=CARTESIAN_POINT('',(0.,63.5,24.75));
#18555=CARTESIAN_POINT('Origin',(0.,31.75,0.));
#18556=CARTESIAN_POINT('',(0.,56.5,-27.5875));
#18557=CARTESIAN_POINT('',(0.,7.,-27.5875));
#18558=CARTESIAN_POINT('',(0.,44.125,-27.5875));
#18559=CARTESIAN_POINT('',(0.,59.3375,-24.75));
#18560=CARTESIAN_POINT('Origin',(0.,56.5,-24.75));
#18561=CARTESIAN_POINT('',(0.,59.3375,24.75));
#18562=CARTESIAN_POINT('',(0.,59.3375,12.375));
#18563=CARTESIAN_POINT('',(0.,56.5,27.5875));
#18564=CARTESIAN_POINT('Origin',(0.,56.5,24.75));
#18565=CARTESIAN_POINT('',(0.,7.,27.5875));
#18566=CARTESIAN_POINT('',(0.,19.375,27.5875));
#18567=CARTESIAN_POINT('',(0.,4.1625,24.75));
#18568=CARTESIAN_POINT('Origin',(0.,7.,24.75));
#18569=CARTESIAN_POINT('',(0.,4.1625,-24.75));
#18570=CARTESIAN_POINT('',(0.,4.1625,-12.375));
#18571=CARTESIAN_POINT('Origin',(0.,7.,-24.75));
#18572=CARTESIAN_POINT('Origin',(0.3,44.125,-27.2875));
#18573=CARTESIAN_POINT('',(0.,7.,-27.5875));
#18574=CARTESIAN_POINT('',(0.6,56.5,-26.9875));
#18575=CARTESIAN_POINT('Origin',(0.3,7.,-24.75));
#18576=CARTESIAN_POINT('',(0.,4.1625,-24.75));
#18577=CARTESIAN_POINT('Origin',(0.3,4.4625,-12.375));
#18578=CARTESIAN_POINT('',(0.6,4.7625,24.75));
#18579=CARTESIAN_POINT('',(0.,4.1625,24.75));
#18580=CARTESIAN_POINT('',(0.6,4.7625,-12.375));
#18581=CARTESIAN_POINT('Origin',(0.3,7.,24.75));
#18582=CARTESIAN_POINT('',(0.6,7.,26.9875));
#18583=CARTESIAN_POINT('',(0.,7.,27.5875));
#18584=CARTESIAN_POINT('Origin',(0.6,7.,24.75));
#18585=CARTESIAN_POINT('Origin',(0.3,19.375,27.2875));
#18586=CARTESIAN_POINT('',(0.6,56.5,26.9875));
#18587=CARTESIAN_POINT('',(0.,56.5,27.5875));
#18588=CARTESIAN_POINT('',(0.6,19.375,26.9875));
#18589=CARTESIAN_POINT('Origin',(0.3,56.5,24.75));
#18590=CARTESIAN_POINT('',(0.,59.3375,24.75));
#18591=CARTESIAN_POINT('Origin',(0.6,56.5,24.75));
#18592=CARTESIAN_POINT('Origin',(0.3,59.0375,12.375));
#18593=CARTESIAN_POINT('',(0.,59.3375,-24.75));
#18594=CARTESIAN_POINT('Origin',(0.3,56.5,-24.75));
#18595=CARTESIAN_POINT('Origin',(0.,56.5,24.75));
#18596=CARTESIAN_POINT('',(0.,56.5,26.9875));
#18597=CARTESIAN_POINT('Origin',(15.2,31.75,-31.75));
#18598=CARTESIAN_POINT('',(10.,31.75,-31.75));
#18599=CARTESIAN_POINT('Origin',(15.2,31.75,-31.75));
#18600=CARTESIAN_POINT('',(10.,31.75,-31.75));
#18601=CARTESIAN_POINT('Origin',(0.,7.,26.9875));
#18602=CARTESIAN_POINT('',(0.,7.,26.9875));
#18603=CARTESIAN_POINT('Origin',(0.,7.,24.75));
#18604=CARTESIAN_POINT('',(0.,4.7625,24.75));
#18605=CARTESIAN_POINT('Origin',(0.,4.7625,-24.75));
#18606=CARTESIAN_POINT('Origin',(0.,63.5,-24.75));
#18607=CARTESIAN_POINT('',(0.,63.5,-24.75));
#18608=CARTESIAN_POINT('Origin',(0.,56.5,-24.75));
#18609=CARTESIAN_POINT('',(0.,56.5,-31.75));
#18610=CARTESIAN_POINT('Origin',(0.,7.,-31.75));
#32279=UNCERTAINTY_MEASURE_WITH_UNIT(LENGTH_MEASURE(0.01),#32310,
'DISTANCE_ACCURACY_VALUE',
'Maximum model space distance between geometric entities at asserted c
onnectivities');
#32293=UNCERTAINTY_MEASURE_WITH_UNIT(LENGTH_MEASURE(0.01),#32310,
'DISTANCE_ACCURACY_VALUE',
'Maximum model space distance between geometric entities at asserted c
onnectivities');
#32295=(
GEOMETRIC_REPRESENTATION_CONTEXT(3)
GLOBAL_UNCERTAINTY_ASSIGNED_CONTEXT((#32279))
GLOBAL_UNIT_ASSIGNED_CONTEXT((#32310,#32312,#32313))
REPRESENTATION_CONTEXT('','3D')
);
#32309=(
GEOMETRIC_REPRESENTATION_CONTEXT(3)
GLOBAL_UNCERTAINTY_ASSIGNED_CONTEXT((#32293))
GLOBAL_UNIT_ASSIGNED_CONTEXT((#32310,#32312,#32313))
REPRESENTATION_CONTEXT('','3D')
);
#32310=(
LENGTH_UNIT()
NAMED_UNIT(*)
SI_UNIT(.MILLI.,.METRE.)
);
#32312=(
NAMED_UNIT(*)
PLANE_ANGLE_UNIT()
SI_UNIT($,.RADIAN.)
);
#32313=(
NAMED_UNIT(*)
SI_UNIT($,.STERADIAN.)
SOLID_ANGLE_UNIT()
);
#32315=SHAPE_DEFINITION_REPRESENTATION(#32330,#32362);
#32330=PRODUCT_DEFINITION_SHAPE('',$,#32378);
#32362=SHAPE_REPRESENTATION('',(#13974),#32295);
#32376=PRODUCT_DEFINITION_CONTEXT('part definition',#32423,'design');
#32378=PRODUCT_DEFINITION('2026-10-25-00-35-15-561',
'01_Outer_Tube_2.5sq_x_3-16',#32393,#32376);
#32393=PRODUCT_DEFINITION_FORMATION('',$,#32426);
#32423=APPLICATION_CONTEXT(
'Core Data for Automotive Mechanical Design Process');
#32424=PRODUCT_CONTEXT('part definition',#32423,'mechanical');
#32426=PRODUCT('2026-10-25-00-35-15-561','01_Outer_Tube_2.5sq_x_3-16',$,
(#32424));
#32482=COLOUR_RGB('Light Blue',0.38,0.62,0.78);
#32483=FILL_AREA_STYLE_COLOUR('',#32482);
#32484=FILL_AREA_STYLE('',(#32483));
#32485=SURFACE_STYLE_FILL_AREA(#32484);
#32486=SURFACE_SIDE_STYLE('',(#32485));
#32487=SURFACE_STYLE_USAGE(.BOTH.,#32486);
#32488=PRESENTATION_STYLE_ASSIGNMENT((#32487));
ENDSEC;
END-ISO-10303-21;
